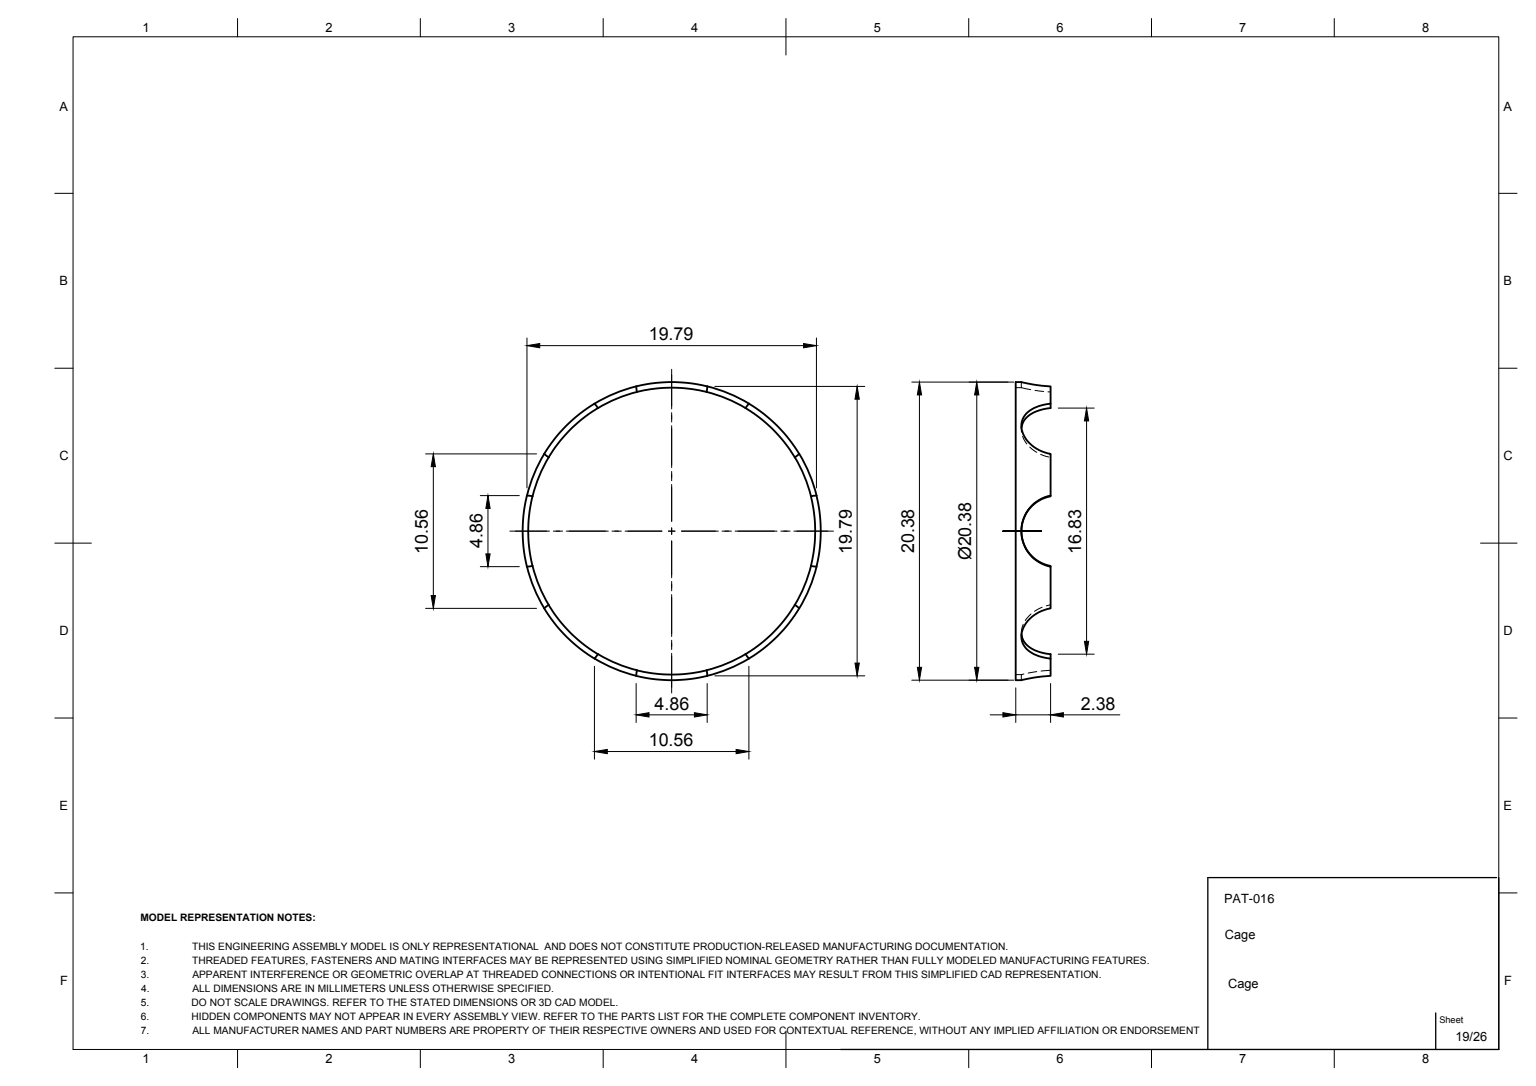
ISO-10303-21;
HEADER;
/* Generated by software containing ST-Developer
 * from STEP Tools, Inc. (www.steptools.com) 
 */

FILE_DESCRIPTION(
/* description */ ('Bracket-mounted idler roller'),
/* implementation_level */ '2;1');

FILE_NAME(
/* name */ 'Cage.step',
/* time_stamp */ '2026-10-28T03:26:42-07:00',
/* author */ (''),
/* organization */ (''),
/* preprocessor_version */ 'ST-DEVELOPER v20.2',
/* originating_system */ 'Autodesk Translation Framework v15.17.0.0',
/* authorisation */ '');

FILE_SCHEMA (('AUTOMOTIVE_DESIGN { 1 0 10303 214 3 1 1 }'));
ENDSEC;

DATA;
#10=MECHANICAL_DESIGN_GEOMETRIC_PRESENTATION_REPRESENTATION('',(#301),#6241);
#187=B_SPLINE_CURVE_WITH_KNOTS('',3,(#5456,#5457,#5458,#5459,#5460,#5461,
#5462,#5463,#5464,#5465,#5466,#5467,#5468,#5469,#5470,#5471,#5472,#5473,
#5474,#5475,#5476,#5477),.UNSPECIFIED.,.F.,.F.,(4,2,2,2,2,2,2,2,2,2,4),
(0.0473477652366656,0.126350602536658,0.189525903804987,0.252701205073317,
0.313298422430275,0.373895639787233,0.434492857144191,0.495090074501149,
0.558265375769478,0.621440677037807,0.7004435143378),.UNSPECIFIED.);
#188=B_SPLINE_CURVE_WITH_KNOTS('',3,(#5481,#5482,#5483,#5484,#5485,#5486,
#5487,#5488,#5489,#5490,#5491,#5492,#5493,#5494,#5495,#5496,#5497,#5498,
#5499,#5500,#5501,#5502),.UNSPECIFIED.,.F.,.F.,(4,2,2,2,2,2,2,2,2,2,4),
(0.0464897534940957,0.0852567806515119,0.170513561303024,0.246687263103517,
0.308657850341199,0.370628437578881,0.432599024816563,0.494569612054245,
0.570743313854739,0.656000094506251,0.694767121663666),.UNSPECIFIED.);
#189=B_SPLINE_CURVE_WITH_KNOTS('',3,(#5508,#5509,#5510,#5511,#5512,#5513,
#5514,#5515,#5516,#5517,#5518,#5519,#5520,#5521,#5522,#5523,#5524,#5525,
#5526,#5527,#5528,#5529),.UNSPECIFIED.,.F.,.F.,(4,2,2,2,2,2,2,2,2,2,4),
(0.0464897534940957,0.0852567806515118,0.170513561303024,0.246687263103517,
0.308657850341199,0.370628437578881,0.432599024816563,0.494569612054245,
0.570743313854738,0.65600009450625,0.694767121663666),.UNSPECIFIED.);
#190=B_SPLINE_CURVE_WITH_KNOTS('',3,(#5533,#5534,#5535,#5536,#5537,#5538,
#5539,#5540,#5541,#5542,#5543,#5544,#5545,#5546,#5547,#5548,#5549,#5550,
#5551,#5552,#5553,#5554),.UNSPECIFIED.,.F.,.F.,(4,2,2,2,2,2,2,2,2,2,4),
(0.0464897534940957,0.0852567806515119,0.170513561303024,0.246687263103517,
0.308657850341199,0.370628437578881,0.432599024816563,0.494569612054245,
0.570743313854739,0.656000094506251,0.694767121663666),.UNSPECIFIED.);
#191=B_SPLINE_CURVE_WITH_KNOTS('',3,(#5558,#5559,#5560,#5561,#5562,#5563,
#5564,#5565,#5566,#5567,#5568,#5569),.UNSPECIFIED.,.F.,.F.,(4,2,2,2,2,4),
(0.0464897534940957,0.0852567806515119,0.170513561303024,0.246687263103517,
0.308657850341199,0.370628437578881),.UNSPECIFIED.);
#192=B_SPLINE_CURVE_WITH_KNOTS('',3,(#5574,#5575,#5576,#5577,#5578,#5579,
#5580,#5581,#5582,#5583,#5584,#5585),.UNSPECIFIED.,.F.,.F.,(4,2,2,2,2,4),
(0.370628437578881,0.432599024816563,0.494569612054245,0.570743313854738,
0.65600009450625,0.694767121663666),.UNSPECIFIED.);
#193=B_SPLINE_CURVE_WITH_KNOTS('',3,(#5589,#5590,#5591,#5592,#5593,#5594,
#5595,#5596,#5597,#5598,#5599,#5600,#5601,#5602,#5603,#5604,#5605,#5606,
#5607,#5608,#5609,#5610),.UNSPECIFIED.,.F.,.F.,(4,2,2,2,2,2,2,2,2,2,4),
(0.0464897534940957,0.0852567806515121,0.170513561303024,0.246687263103518,
0.308657850341199,0.370628437578881,0.432599024816563,0.494569612054245,
0.570743313854738,0.65600009450625,0.694767121663666),.UNSPECIFIED.);
#194=B_SPLINE_CURVE_WITH_KNOTS('',3,(#5614,#5615,#5616,#5617,#5618,#5619,
#5620,#5621,#5622,#5623,#5624,#5625,#5626,#5627,#5628,#5629,#5630,#5631,
#5632,#5633,#5634,#5635),.UNSPECIFIED.,.F.,.F.,(4,2,2,2,2,2,2,2,2,2,4),
(0.0464897534940957,0.0852567806515119,0.170513561303024,0.246687263103517,
0.308657850341199,0.370628437578881,0.432599024816563,0.494569612054245,
0.570743313854738,0.65600009450625,0.694767121663667),.UNSPECIFIED.);
#195=B_SPLINE_CURVE_WITH_KNOTS('',3,(#5639,#5640,#5641,#5642,#5643,#5644,
#5645,#5646,#5647,#5648,#5649,#5650,#5651,#5652,#5653,#5654,#5655,#5656,
#5657,#5658,#5659,#5660),.UNSPECIFIED.,.F.,.F.,(4,2,2,2,2,2,2,2,2,2,4),
(0.0464897534940957,0.0852567806515119,0.170513561303024,0.246687263103517,
0.308657850341199,0.370628437578881,0.432599024816563,0.494569612054245,
0.570743313854738,0.65600009450625,0.694767121663666),.UNSPECIFIED.);
#196=B_SPLINE_CURVE_WITH_KNOTS('',3,(#5664,#5665,#5666,#5667,#5668,#5669,
#5670,#5671,#5672,#5673,#5674,#5675,#5676,#5677,#5678,#5679,#5680,#5681,
#5682,#5683,#5684,#5685),.UNSPECIFIED.,.F.,.F.,(4,2,2,2,2,2,2,2,2,2,4),
(0.0464897534940957,0.0852567806515119,0.170513561303024,0.246687263103517,
0.308657850341199,0.370628437578881,0.432599024816563,0.494569612054245,
0.570743313854739,0.656000094506251,0.694767121663667),.UNSPECIFIED.);
#197=B_SPLINE_CURVE_WITH_KNOTS('',3,(#5693,#5694,#5695,#5696,#5697,#5698,
#5699,#5700,#5701,#5702,#5703,#5704,#5705,#5706,#5707,#5708,#5709,#5710,
#5711,#5712,#5713,#5714),.UNSPECIFIED.,.F.,.F.,(4,2,2,2,2,2,2,2,2,2,4),
(0.0473477652366656,0.126350602536658,0.189525903804987,0.252701205073316,
0.313298422430274,0.373895639787232,0.434492857144191,0.495090074501149,
0.558265375769478,0.621440677037807,0.7004435143378),.UNSPECIFIED.);
#198=B_SPLINE_CURVE_WITH_KNOTS('',3,(#5722,#5723,#5724,#5725,#5726,#5727,
#5728,#5729,#5730,#5731,#5732,#5733,#5734,#5735,#5736,#5737,#5738,#5739,
#5740,#5741,#5742,#5743),.UNSPECIFIED.,.F.,.F.,(4,2,2,2,2,2,2,2,2,2,4),
(0.0473477652366656,0.126350602536658,0.189525903804987,0.252701205073317,
0.313298422430275,0.373895639787233,0.434492857144191,0.495090074501149,
0.558265375769478,0.621440677037807,0.7004435143378),.UNSPECIFIED.);
#199=B_SPLINE_CURVE_WITH_KNOTS('',3,(#5752,#5753,#5754,#5755,#5756,#5757,
#5758,#5759,#5760,#5761,#5762,#5763),.UNSPECIFIED.,.F.,.F.,(4,2,2,2,2,4),
(0.0473477652366656,0.126350602536658,0.189525903804987,0.252701205073316,
0.313298422430275,0.373895639787233),.UNSPECIFIED.);
#200=B_SPLINE_CURVE_WITH_KNOTS('',3,(#5765,#5766,#5767,#5768,#5769,#5770,
#5771,#5772,#5773,#5774,#5775,#5776),.UNSPECIFIED.,.F.,.F.,(4,2,2,2,2,4),
(0.373895639787233,0.434492857144191,0.495090074501149,0.558265375769478,
0.621440677037807,0.7004435143378),.UNSPECIFIED.);
#201=B_SPLINE_CURVE_WITH_KNOTS('',3,(#5783,#5784,#5785,#5786,#5787,#5788,
#5789,#5790,#5791,#5792,#5793,#5794,#5795,#5796,#5797,#5798,#5799,#5800,
#5801,#5802,#5803,#5804),.UNSPECIFIED.,.F.,.F.,(4,2,2,2,2,2,2,2,2,2,4),
(0.0473477652366656,0.126350602536658,0.189525903804987,0.252701205073316,
0.313298422430275,0.373895639787233,0.434492857144191,0.495090074501149,
0.558265375769478,0.621440677037807,0.7004435143378),.UNSPECIFIED.);
#202=B_SPLINE_CURVE_WITH_KNOTS('',3,(#5812,#5813,#5814,#5815,#5816,#5817,
#5818,#5819,#5820,#5821,#5822,#5823,#5824,#5825,#5826,#5827,#5828,#5829,
#5830,#5831,#5832,#5833),.UNSPECIFIED.,.F.,.F.,(4,2,2,2,2,2,2,2,2,2,4),
(0.0473477652366656,0.126350602536658,0.189525903804987,0.252701205073317,
0.313298422430275,0.373895639787233,0.434492857144191,0.495090074501149,
0.558265375769478,0.621440677037807,0.7004435143378),.UNSPECIFIED.);
#203=B_SPLINE_CURVE_WITH_KNOTS('',3,(#5841,#5842,#5843,#5844,#5845,#5846,
#5847,#5848,#5849,#5850,#5851,#5852,#5853,#5854,#5855,#5856,#5857,#5858,
#5859,#5860,#5861,#5862),.UNSPECIFIED.,.F.,.F.,(4,2,2,2,2,2,2,2,2,2,4),
(0.0473477652366656,0.126350602536658,0.189525903804987,0.252701205073316,
0.313298422430275,0.373895639787233,0.434492857144191,0.495090074501149,
0.558265375769478,0.621440677037807,0.7004435143378),.UNSPECIFIED.);
#204=B_SPLINE_CURVE_WITH_KNOTS('',3,(#5871,#5872,#5873,#5874,#5875,#5876,
#5877,#5878,#5879,#5880,#5881,#5882,#5883,#5884,#5885,#5886,#5887,#5888,
#5889,#5890,#5891,#5892),.UNSPECIFIED.,.F.,.F.,(4,2,2,2,2,2,2,2,2,2,4),
(0.0473477652366656,0.126350602536658,0.189525903804987,0.252701205073317,
0.313298422430275,0.373895639787233,0.434492857144191,0.495090074501149,
0.558265375769478,0.621440677037807,0.7004435143378),.UNSPECIFIED.);
#213=SPHERICAL_SURFACE('',#3665,0.247676);
#214=SPHERICAL_SURFACE('',#3681,0.247676);
#215=SPHERICAL_SURFACE('',#3686,0.247676);
#216=SPHERICAL_SURFACE('',#3691,0.247676);
#217=SPHERICAL_SURFACE('',#3696,0.247676);
#218=SPHERICAL_SURFACE('',#3701,0.247676);
#219=SPHERICAL_SURFACE('',#3706,0.247676);
#220=SPHERICAL_SURFACE('',#3714,0.247676);
#252=SHAPE_REPRESENTATION_RELATIONSHIP('SRR','None',#6357,#273);
#273=ADVANCED_BREP_SHAPE_REPRESENTATION('',(#329),#6233);
#301=STYLED_ITEM('',(#6538),#329);
#329=MANIFOLD_SOLID_BREP('Continuous crown cage',#3204);
#377=FACE_BOUND('',#881,.T.);
#482=PLANE('',#3678);
#483=PLANE('',#3683);
#484=PLANE('',#3688);
#485=PLANE('',#3693);
#486=PLANE('',#3698);
#487=PLANE('',#3703);
#488=PLANE('',#3712);
#489=PLANE('',#3716);
#490=PLANE('',#3717);
#631=FACE_OUTER_BOUND('',#863,.T.);
#632=FACE_OUTER_BOUND('',#864,.T.);
#633=FACE_OUTER_BOUND('',#865,.T.);
#634=FACE_OUTER_BOUND('',#866,.T.);
#635=FACE_OUTER_BOUND('',#867,.T.);
#636=FACE_OUTER_BOUND('',#868,.T.);
#637=FACE_OUTER_BOUND('',#869,.T.);
#638=FACE_OUTER_BOUND('',#870,.T.);
#639=FACE_OUTER_BOUND('',#871,.T.);
#640=FACE_OUTER_BOUND('',#872,.T.);
#641=FACE_OUTER_BOUND('',#873,.T.);
#642=FACE_OUTER_BOUND('',#874,.T.);
#643=FACE_OUTER_BOUND('',#875,.T.);
#644=FACE_OUTER_BOUND('',#876,.T.);
#645=FACE_OUTER_BOUND('',#877,.T.);
#646=FACE_OUTER_BOUND('',#878,.T.);
#647=FACE_OUTER_BOUND('',#879,.T.);
#648=FACE_OUTER_BOUND('',#880,.T.);
#649=FACE_OUTER_BOUND('',#882,.T.);
#863=EDGE_LOOP('',(#2600,#2601,#2602,#2603));
#864=EDGE_LOOP('',(#2604,#2605,#2606,#2607,#2608,#2609,#2610,#2611,#2612,
#2613,#2614,#2615,#2616,#2617,#2618,#2619,#2620,#2621,#2622,#2623));
#865=EDGE_LOOP('',(#2624,#2625,#2626,#2627));
#866=EDGE_LOOP('',(#2628,#2629,#2630,#2631));
#867=EDGE_LOOP('',(#2632,#2633,#2634,#2635));
#868=EDGE_LOOP('',(#2636,#2637,#2638,#2639));
#869=EDGE_LOOP('',(#2640,#2641,#2642,#2643));
#870=EDGE_LOOP('',(#2644,#2645,#2646,#2647,#2648,#2649));
#871=EDGE_LOOP('',(#2650,#2651,#2652,#2653));
#872=EDGE_LOOP('',(#2654,#2655,#2656,#2657));
#873=EDGE_LOOP('',(#2658,#2659,#2660,#2661));
#874=EDGE_LOOP('',(#2662,#2663,#2664,#2665));
#875=EDGE_LOOP('',(#2666,#2667,#2668,#2669));
#876=EDGE_LOOP('',(#2670,#2671,#2672,#2673));
#877=EDGE_LOOP('',(#2674,#2675,#2676,#2677,#2678,#2679,#2680,#2681,#2682,
#2683,#2684,#2685,#2686,#2687,#2688,#2689,#2690,#2691,#2692,#2693));
#878=EDGE_LOOP('',(#2694,#2695,#2696,#2697));
#879=EDGE_LOOP('',(#2698,#2699,#2700,#2701));
#880=EDGE_LOOP('',(#2702));
#881=EDGE_LOOP('',(#2703));
#882=EDGE_LOOP('',(#2704,#2705,#2706,#2707));
#1109=LINE('',#5571,#1291);
#1110=LINE('',#5867,#1292);
#1291=VECTOR('',#4470,1.019052);
#1292=VECTOR('',#4547,0.980948);
#1430=CIRCLE('',#3666,0.243053047864041);
#1431=CIRCLE('',#3667,0.243053047864041);
#1432=CIRCLE('',#3669,1.019052);
#1433=CIRCLE('',#3670,1.019052);
#1434=CIRCLE('',#3671,1.019052);
#1435=CIRCLE('',#3672,1.019052);
#1436=CIRCLE('',#3673,1.019052);
#1437=CIRCLE('',#3674,1.019052);
#1438=CIRCLE('',#3675,1.019052);
#1439=CIRCLE('',#3676,1.019052);
#1440=CIRCLE('',#3677,1.019052);
#1441=CIRCLE('',#3679,0.980948);
#1442=CIRCLE('',#3680,0.243053047864041);
#1443=CIRCLE('',#3682,0.243053047864041);
#1444=CIRCLE('',#3684,0.980948);
#1445=CIRCLE('',#3685,0.243053047864041);
#1446=CIRCLE('',#3687,0.243053047864041);
#1447=CIRCLE('',#3689,0.980948);
#1448=CIRCLE('',#3690,0.243053047864041);
#1449=CIRCLE('',#3692,0.243053047864041);
#1450=CIRCLE('',#3694,0.980948);
#1451=CIRCLE('',#3695,0.243053047864041);
#1452=CIRCLE('',#3697,0.243053047864041);
#1453=CIRCLE('',#3699,0.980948);
#1454=CIRCLE('',#3700,0.243053047864041);
#1455=CIRCLE('',#3702,0.243053047864041);
#1456=CIRCLE('',#3704,0.980948);
#1457=CIRCLE('',#3705,0.243053047864041);
#1458=CIRCLE('',#3707,0.243053047864041);
#1459=CIRCLE('',#3709,0.980948);
#1460=CIRCLE('',#3710,0.980948);
#1461=CIRCLE('',#3711,0.980948);
#1462=CIRCLE('',#3713,0.243053047864041);
#1463=CIRCLE('',#3715,0.243053047864041);
#1677=VERTEX_POINT('',#5454);
#1678=VERTEX_POINT('',#5455);
#1679=VERTEX_POINT('',#5478);
#1680=VERTEX_POINT('',#5480);
#1681=VERTEX_POINT('',#5505);
#1682=VERTEX_POINT('',#5507);
#1683=VERTEX_POINT('',#5530);
#1684=VERTEX_POINT('',#5532);
#1685=VERTEX_POINT('',#5555);
#1686=VERTEX_POINT('',#5557);
#1687=VERTEX_POINT('',#5570);
#1688=VERTEX_POINT('',#5573);
#1689=VERTEX_POINT('',#5586);
#1690=VERTEX_POINT('',#5588);
#1691=VERTEX_POINT('',#5611);
#1692=VERTEX_POINT('',#5613);
#1693=VERTEX_POINT('',#5636);
#1694=VERTEX_POINT('',#5638);
#1695=VERTEX_POINT('',#5661);
#1696=VERTEX_POINT('',#5663);
#1697=VERTEX_POINT('',#5688);
#1698=VERTEX_POINT('',#5692);
#1699=VERTEX_POINT('',#5717);
#1700=VERTEX_POINT('',#5721);
#1701=VERTEX_POINT('',#5746);
#1702=VERTEX_POINT('',#5750);
#1703=VERTEX_POINT('',#5751);
#1704=VERTEX_POINT('',#5778);
#1705=VERTEX_POINT('',#5782);
#1706=VERTEX_POINT('',#5807);
#1707=VERTEX_POINT('',#5811);
#1708=VERTEX_POINT('',#5836);
#1709=VERTEX_POINT('',#5840);
#1710=VERTEX_POINT('',#5865);
#1711=VERTEX_POINT('',#5868);
#1712=VERTEX_POINT('',#5870);
#2002=EDGE_CURVE('',#1677,#1678,#187,.T.);
#2003=EDGE_CURVE('',#1679,#1677,#1430,.T.);
#2004=EDGE_CURVE('',#1680,#1679,#188,.T.);
#2005=EDGE_CURVE('',#1678,#1680,#1431,.T.);
#2006=EDGE_CURVE('',#1681,#1679,#1432,.T.);
#2007=EDGE_CURVE('',#1681,#1682,#189,.T.);
#2008=EDGE_CURVE('',#1683,#1682,#1433,.T.);
#2009=EDGE_CURVE('',#1683,#1684,#190,.T.);
#2010=EDGE_CURVE('',#1685,#1684,#1434,.T.);
#2011=EDGE_CURVE('',#1685,#1686,#191,.T.);
#2012=EDGE_CURVE('',#1686,#1687,#1109,.T.);
#2013=EDGE_CURVE('',#1687,#1687,#1435,.T.);
#2014=EDGE_CURVE('',#1686,#1688,#192,.T.);
#2015=EDGE_CURVE('',#1689,#1688,#1436,.T.);
#2016=EDGE_CURVE('',#1689,#1690,#193,.T.);
#2017=EDGE_CURVE('',#1691,#1690,#1437,.T.);
#2018=EDGE_CURVE('',#1691,#1692,#194,.T.);
#2019=EDGE_CURVE('',#1693,#1692,#1438,.T.);
#2020=EDGE_CURVE('',#1693,#1694,#195,.T.);
#2021=EDGE_CURVE('',#1695,#1694,#1439,.T.);
#2022=EDGE_CURVE('',#1695,#1696,#196,.T.);
#2023=EDGE_CURVE('',#1680,#1696,#1440,.T.);
#2024=EDGE_CURVE('',#1677,#1697,#1441,.T.);
#2025=EDGE_CURVE('',#1697,#1681,#1442,.T.);
#2026=EDGE_CURVE('',#1698,#1697,#197,.T.);
#2027=EDGE_CURVE('',#1682,#1698,#1443,.T.);
#2028=EDGE_CURVE('',#1698,#1699,#1444,.T.);
#2029=EDGE_CURVE('',#1699,#1683,#1445,.T.);
#2030=EDGE_CURVE('',#1700,#1699,#198,.T.);
#2031=EDGE_CURVE('',#1684,#1700,#1446,.T.);
#2032=EDGE_CURVE('',#1700,#1701,#1447,.T.);
#2033=EDGE_CURVE('',#1701,#1685,#1448,.T.);
#2034=EDGE_CURVE('',#1702,#1703,#199,.T.);
#2035=EDGE_CURVE('',#1688,#1702,#1449,.T.);
#2036=EDGE_CURVE('',#1703,#1701,#200,.T.);
#2037=EDGE_CURVE('',#1702,#1704,#1450,.T.);
#2038=EDGE_CURVE('',#1704,#1689,#1451,.T.);
#2039=EDGE_CURVE('',#1705,#1704,#201,.T.);
#2040=EDGE_CURVE('',#1690,#1705,#1452,.T.);
#2041=EDGE_CURVE('',#1705,#1706,#1453,.T.);
#2042=EDGE_CURVE('',#1706,#1691,#1454,.T.);
#2043=EDGE_CURVE('',#1707,#1706,#202,.T.);
#2044=EDGE_CURVE('',#1692,#1707,#1455,.T.);
#2045=EDGE_CURVE('',#1707,#1708,#1456,.T.);
#2046=EDGE_CURVE('',#1708,#1693,#1457,.T.);
#2047=EDGE_CURVE('',#1709,#1708,#203,.T.);
#2048=EDGE_CURVE('',#1694,#1709,#1458,.T.);
#2049=EDGE_CURVE('',#1710,#1710,#1459,.T.);
#2050=EDGE_CURVE('',#1710,#1703,#1110,.T.);
#2051=EDGE_CURVE('',#1711,#1678,#1460,.T.);
#2052=EDGE_CURVE('',#1711,#1712,#204,.T.);
#2053=EDGE_CURVE('',#1709,#1712,#1461,.T.);
#2054=EDGE_CURVE('',#1696,#1711,#1462,.T.);
#2055=EDGE_CURVE('',#1712,#1695,#1463,.T.);
#2600=ORIENTED_EDGE('',*,*,#2002,.F.);
#2601=ORIENTED_EDGE('',*,*,#2003,.F.);
#2602=ORIENTED_EDGE('',*,*,#2004,.F.);
#2603=ORIENTED_EDGE('',*,*,#2005,.F.);
#2604=ORIENTED_EDGE('',*,*,#2004,.T.);
#2605=ORIENTED_EDGE('',*,*,#2006,.F.);
#2606=ORIENTED_EDGE('',*,*,#2007,.T.);
#2607=ORIENTED_EDGE('',*,*,#2008,.F.);
#2608=ORIENTED_EDGE('',*,*,#2009,.T.);
#2609=ORIENTED_EDGE('',*,*,#2010,.F.);
#2610=ORIENTED_EDGE('',*,*,#2011,.T.);
#2611=ORIENTED_EDGE('',*,*,#2012,.T.);
#2612=ORIENTED_EDGE('',*,*,#2013,.F.);
#2613=ORIENTED_EDGE('',*,*,#2012,.F.);
#2614=ORIENTED_EDGE('',*,*,#2014,.T.);
#2615=ORIENTED_EDGE('',*,*,#2015,.F.);
#2616=ORIENTED_EDGE('',*,*,#2016,.T.);
#2617=ORIENTED_EDGE('',*,*,#2017,.F.);
#2618=ORIENTED_EDGE('',*,*,#2018,.T.);
#2619=ORIENTED_EDGE('',*,*,#2019,.F.);
#2620=ORIENTED_EDGE('',*,*,#2020,.T.);
#2621=ORIENTED_EDGE('',*,*,#2021,.F.);
#2622=ORIENTED_EDGE('',*,*,#2022,.T.);
#2623=ORIENTED_EDGE('',*,*,#2023,.F.);
#2624=ORIENTED_EDGE('',*,*,#2003,.T.);
#2625=ORIENTED_EDGE('',*,*,#2024,.T.);
#2626=ORIENTED_EDGE('',*,*,#2025,.T.);
#2627=ORIENTED_EDGE('',*,*,#2006,.T.);
#2628=ORIENTED_EDGE('',*,*,#2026,.F.);
#2629=ORIENTED_EDGE('',*,*,#2027,.F.);
#2630=ORIENTED_EDGE('',*,*,#2007,.F.);
#2631=ORIENTED_EDGE('',*,*,#2025,.F.);
#2632=ORIENTED_EDGE('',*,*,#2027,.T.);
#2633=ORIENTED_EDGE('',*,*,#2028,.T.);
#2634=ORIENTED_EDGE('',*,*,#2029,.T.);
#2635=ORIENTED_EDGE('',*,*,#2008,.T.);
#2636=ORIENTED_EDGE('',*,*,#2030,.F.);
#2637=ORIENTED_EDGE('',*,*,#2031,.F.);
#2638=ORIENTED_EDGE('',*,*,#2009,.F.);
#2639=ORIENTED_EDGE('',*,*,#2029,.F.);
#2640=ORIENTED_EDGE('',*,*,#2031,.T.);
#2641=ORIENTED_EDGE('',*,*,#2032,.T.);
#2642=ORIENTED_EDGE('',*,*,#2033,.T.);
#2643=ORIENTED_EDGE('',*,*,#2010,.T.);
#2644=ORIENTED_EDGE('',*,*,#2034,.F.);
#2645=ORIENTED_EDGE('',*,*,#2035,.F.);
#2646=ORIENTED_EDGE('',*,*,#2014,.F.);
#2647=ORIENTED_EDGE('',*,*,#2011,.F.);
#2648=ORIENTED_EDGE('',*,*,#2033,.F.);
#2649=ORIENTED_EDGE('',*,*,#2036,.F.);
#2650=ORIENTED_EDGE('',*,*,#2035,.T.);
#2651=ORIENTED_EDGE('',*,*,#2037,.T.);
#2652=ORIENTED_EDGE('',*,*,#2038,.T.);
#2653=ORIENTED_EDGE('',*,*,#2015,.T.);
#2654=ORIENTED_EDGE('',*,*,#2039,.F.);
#2655=ORIENTED_EDGE('',*,*,#2040,.F.);
#2656=ORIENTED_EDGE('',*,*,#2016,.F.);
#2657=ORIENTED_EDGE('',*,*,#2038,.F.);
#2658=ORIENTED_EDGE('',*,*,#2040,.T.);
#2659=ORIENTED_EDGE('',*,*,#2041,.T.);
#2660=ORIENTED_EDGE('',*,*,#2042,.T.);
#2661=ORIENTED_EDGE('',*,*,#2017,.T.);
#2662=ORIENTED_EDGE('',*,*,#2043,.F.);
#2663=ORIENTED_EDGE('',*,*,#2044,.F.);
#2664=ORIENTED_EDGE('',*,*,#2018,.F.);
#2665=ORIENTED_EDGE('',*,*,#2042,.F.);
#2666=ORIENTED_EDGE('',*,*,#2044,.T.);
#2667=ORIENTED_EDGE('',*,*,#2045,.T.);
#2668=ORIENTED_EDGE('',*,*,#2046,.T.);
#2669=ORIENTED_EDGE('',*,*,#2019,.T.);
#2670=ORIENTED_EDGE('',*,*,#2020,.F.);
#2671=ORIENTED_EDGE('',*,*,#2046,.F.);
#2672=ORIENTED_EDGE('',*,*,#2047,.F.);
#2673=ORIENTED_EDGE('',*,*,#2048,.F.);
#2674=ORIENTED_EDGE('',*,*,#2049,.F.);
#2675=ORIENTED_EDGE('',*,*,#2050,.T.);
#2676=ORIENTED_EDGE('',*,*,#2036,.T.);
#2677=ORIENTED_EDGE('',*,*,#2032,.F.);
#2678=ORIENTED_EDGE('',*,*,#2030,.T.);
#2679=ORIENTED_EDGE('',*,*,#2028,.F.);
#2680=ORIENTED_EDGE('',*,*,#2026,.T.);
#2681=ORIENTED_EDGE('',*,*,#2024,.F.);
#2682=ORIENTED_EDGE('',*,*,#2002,.T.);
#2683=ORIENTED_EDGE('',*,*,#2051,.F.);
#2684=ORIENTED_EDGE('',*,*,#2052,.T.);
#2685=ORIENTED_EDGE('',*,*,#2053,.F.);
#2686=ORIENTED_EDGE('',*,*,#2047,.T.);
#2687=ORIENTED_EDGE('',*,*,#2045,.F.);
#2688=ORIENTED_EDGE('',*,*,#2043,.T.);
#2689=ORIENTED_EDGE('',*,*,#2041,.F.);
#2690=ORIENTED_EDGE('',*,*,#2039,.T.);
#2691=ORIENTED_EDGE('',*,*,#2037,.F.);
#2692=ORIENTED_EDGE('',*,*,#2034,.T.);
#2693=ORIENTED_EDGE('',*,*,#2050,.F.);
#2694=ORIENTED_EDGE('',*,*,#2005,.T.);
#2695=ORIENTED_EDGE('',*,*,#2023,.T.);
#2696=ORIENTED_EDGE('',*,*,#2054,.T.);
#2697=ORIENTED_EDGE('',*,*,#2051,.T.);
#2698=ORIENTED_EDGE('',*,*,#2022,.F.);
#2699=ORIENTED_EDGE('',*,*,#2055,.F.);
#2700=ORIENTED_EDGE('',*,*,#2052,.F.);
#2701=ORIENTED_EDGE('',*,*,#2054,.F.);
#2702=ORIENTED_EDGE('',*,*,#2013,.T.);
#2703=ORIENTED_EDGE('',*,*,#2049,.T.);
#2704=ORIENTED_EDGE('',*,*,#2048,.T.);
#2705=ORIENTED_EDGE('',*,*,#2053,.T.);
#2706=ORIENTED_EDGE('',*,*,#2055,.T.);
#2707=ORIENTED_EDGE('',*,*,#2021,.T.);
#2961=CYLINDRICAL_SURFACE('',#3668,1.019052);
#2962=CYLINDRICAL_SURFACE('',#3708,0.980948);
#3106=ADVANCED_FACE('',(#631),#213,.F.);
#3107=ADVANCED_FACE('',(#632),#2961,.T.);
#3108=ADVANCED_FACE('',(#633),#482,.T.);
#3109=ADVANCED_FACE('',(#634),#214,.F.);
#3110=ADVANCED_FACE('',(#635),#483,.T.);
#3111=ADVANCED_FACE('',(#636),#215,.F.);
#3112=ADVANCED_FACE('',(#637),#484,.T.);
#3113=ADVANCED_FACE('',(#638),#216,.F.);
#3114=ADVANCED_FACE('',(#639),#485,.T.);
#3115=ADVANCED_FACE('',(#640),#217,.F.);
#3116=ADVANCED_FACE('',(#641),#486,.T.);
#3117=ADVANCED_FACE('',(#642),#218,.F.);
#3118=ADVANCED_FACE('',(#643),#487,.T.);
#3119=ADVANCED_FACE('',(#644),#219,.F.);
#3120=ADVANCED_FACE('',(#645),#2962,.F.);
#3121=ADVANCED_FACE('',(#646),#488,.T.);
#3122=ADVANCED_FACE('',(#647),#220,.F.);
#3123=ADVANCED_FACE('',(#648,#377),#489,.T.);
#3124=ADVANCED_FACE('',(#649),#490,.T.);
#3204=CLOSED_SHELL('',(#3106,#3107,#3108,#3109,#3110,#3111,#3112,#3113,
#3114,#3115,#3116,#3117,#3118,#3119,#3120,#3121,#3122,#3123,#3124));
#3664=AXIS2_PLACEMENT_3D('',#5452,#4454,#4455);
#3665=AXIS2_PLACEMENT_3D('',#5453,#4456,#4457);
#3666=AXIS2_PLACEMENT_3D('',#5479,#4458,#4459);
#3667=AXIS2_PLACEMENT_3D('',#5503,#4460,#4461);
#3668=AXIS2_PLACEMENT_3D('',#5504,#4462,#4463);
#3669=AXIS2_PLACEMENT_3D('',#5506,#4464,#4465);
#3670=AXIS2_PLACEMENT_3D('',#5531,#4466,#4467);
#3671=AXIS2_PLACEMENT_3D('',#5556,#4468,#4469);
#3672=AXIS2_PLACEMENT_3D('',#5572,#4471,#4472);
#3673=AXIS2_PLACEMENT_3D('',#5587,#4473,#4474);
#3674=AXIS2_PLACEMENT_3D('',#5612,#4475,#4476);
#3675=AXIS2_PLACEMENT_3D('',#5637,#4477,#4478);
#3676=AXIS2_PLACEMENT_3D('',#5662,#4479,#4480);
#3677=AXIS2_PLACEMENT_3D('',#5686,#4481,#4482);
#3678=AXIS2_PLACEMENT_3D('',#5687,#4483,#4484);
#3679=AXIS2_PLACEMENT_3D('',#5689,#4485,#4486);
#3680=AXIS2_PLACEMENT_3D('',#5690,#4487,#4488);
#3681=AXIS2_PLACEMENT_3D('',#5691,#4489,#4490);
#3682=AXIS2_PLACEMENT_3D('',#5715,#4491,#4492);
#3683=AXIS2_PLACEMENT_3D('',#5716,#4493,#4494);
#3684=AXIS2_PLACEMENT_3D('',#5718,#4495,#4496);
#3685=AXIS2_PLACEMENT_3D('',#5719,#4497,#4498);
#3686=AXIS2_PLACEMENT_3D('',#5720,#4499,#4500);
#3687=AXIS2_PLACEMENT_3D('',#5744,#4501,#4502);
#3688=AXIS2_PLACEMENT_3D('',#5745,#4503,#4504);
#3689=AXIS2_PLACEMENT_3D('',#5747,#4505,#4506);
#3690=AXIS2_PLACEMENT_3D('',#5748,#4507,#4508);
#3691=AXIS2_PLACEMENT_3D('',#5749,#4509,#4510);
#3692=AXIS2_PLACEMENT_3D('',#5764,#4511,#4512);
#3693=AXIS2_PLACEMENT_3D('',#5777,#4513,#4514);
#3694=AXIS2_PLACEMENT_3D('',#5779,#4515,#4516);
#3695=AXIS2_PLACEMENT_3D('',#5780,#4517,#4518);
#3696=AXIS2_PLACEMENT_3D('',#5781,#4519,#4520);
#3697=AXIS2_PLACEMENT_3D('',#5805,#4521,#4522);
#3698=AXIS2_PLACEMENT_3D('',#5806,#4523,#4524);
#3699=AXIS2_PLACEMENT_3D('',#5808,#4525,#4526);
#3700=AXIS2_PLACEMENT_3D('',#5809,#4527,#4528);
#3701=AXIS2_PLACEMENT_3D('',#5810,#4529,#4530);
#3702=AXIS2_PLACEMENT_3D('',#5834,#4531,#4532);
#3703=AXIS2_PLACEMENT_3D('',#5835,#4533,#4534);
#3704=AXIS2_PLACEMENT_3D('',#5837,#4535,#4536);
#3705=AXIS2_PLACEMENT_3D('',#5838,#4537,#4538);
#3706=AXIS2_PLACEMENT_3D('',#5839,#4539,#4540);
#3707=AXIS2_PLACEMENT_3D('',#5863,#4541,#4542);
#3708=AXIS2_PLACEMENT_3D('',#5864,#4543,#4544);
#3709=AXIS2_PLACEMENT_3D('',#5866,#4545,#4546);
#3710=AXIS2_PLACEMENT_3D('',#5869,#4548,#4549);
#3711=AXIS2_PLACEMENT_3D('',#5893,#4550,#4551);
#3712=AXIS2_PLACEMENT_3D('',#5894,#4552,#4553);
#3713=AXIS2_PLACEMENT_3D('',#5895,#4554,#4555);
#3714=AXIS2_PLACEMENT_3D('',#5896,#4556,#4557);
#3715=AXIS2_PLACEMENT_3D('',#5897,#4558,#4559);
#3716=AXIS2_PLACEMENT_3D('',#5898,#4560,#4561);
#3717=AXIS2_PLACEMENT_3D('',#5899,#4562,#4563);
#4454=DIRECTION('axis',(0.,0.,1.));
#4455=DIRECTION('refdir',(1.,0.,0.));
#4456=DIRECTION('center_axis',(0.,0.,1.));
#4457=DIRECTION('ref_axis',(1.,0.,0.));
#4458=DIRECTION('center_axis',(0.,-1.,0.));
#4459=DIRECTION('ref_axis',(0.,0.,-1.));
#4460=DIRECTION('center_axis',(0.,-1.,0.));
#4461=DIRECTION('ref_axis',(0.,0.,-1.));
#4462=DIRECTION('center_axis',(0.,1.,0.));
#4463=DIRECTION('ref_axis',(1.,0.,0.));
#4464=DIRECTION('center_axis',(0.,1.,0.));
#4465=DIRECTION('ref_axis',(1.,0.,0.));
#4466=DIRECTION('center_axis',(0.,1.,0.));
#4467=DIRECTION('ref_axis',(1.,0.,0.));
#4468=DIRECTION('center_axis',(0.,1.,0.));
#4469=DIRECTION('ref_axis',(1.,0.,0.));
#4470=DIRECTION('',(0.,-1.,0.));
#4471=DIRECTION('center_axis',(0.,-1.,0.));
#4472=DIRECTION('ref_axis',(1.,0.,0.));
#4473=DIRECTION('center_axis',(0.,1.,0.));
#4474=DIRECTION('ref_axis',(1.,0.,0.));
#4475=DIRECTION('center_axis',(0.,1.,0.));
#4476=DIRECTION('ref_axis',(1.,0.,0.));
#4477=DIRECTION('center_axis',(0.,1.,0.));
#4478=DIRECTION('ref_axis',(1.,0.,0.));
#4479=DIRECTION('center_axis',(0.,1.,0.));
#4480=DIRECTION('ref_axis',(1.,0.,0.));
#4481=DIRECTION('center_axis',(0.,1.,0.));
#4482=DIRECTION('ref_axis',(1.,0.,0.));
#4483=DIRECTION('center_axis',(0.,1.,0.));
#4484=DIRECTION('ref_axis',(1.,0.,0.));
#4485=DIRECTION('center_axis',(0.,-1.,0.));
#4486=DIRECTION('ref_axis',(1.,0.,0.));
#4487=DIRECTION('center_axis',(0.,-1.,0.));
#4488=DIRECTION('ref_axis',(0.,0.,-1.));
#4489=DIRECTION('center_axis',(6.12323399573677E-17,0.,1.));
#4490=DIRECTION('ref_axis',(1.,0.,0.));
#4491=DIRECTION('center_axis',(0.,-1.,0.));
#4492=DIRECTION('ref_axis',(0.,0.,-1.));
#4493=DIRECTION('center_axis',(0.,1.,0.));
#4494=DIRECTION('ref_axis',(1.,0.,0.));
#4495=DIRECTION('center_axis',(0.,-1.,0.));
#4496=DIRECTION('ref_axis',(1.,0.,0.));
#4497=DIRECTION('center_axis',(0.,-1.,0.));
#4498=DIRECTION('ref_axis',(0.,0.,-1.));
#4499=DIRECTION('center_axis',(0.,0.,1.));
#4500=DIRECTION('ref_axis',(1.,0.,0.));
#4501=DIRECTION('center_axis',(0.,-1.,0.));
#4502=DIRECTION('ref_axis',(0.,0.,-1.));
#4503=DIRECTION('center_axis',(0.,1.,0.));
#4504=DIRECTION('ref_axis',(1.,0.,0.));
#4505=DIRECTION('center_axis',(0.,-1.,0.));
#4506=DIRECTION('ref_axis',(1.,0.,0.));
#4507=DIRECTION('center_axis',(0.,-1.,0.));
#4508=DIRECTION('ref_axis',(0.,0.,-1.));
#4509=DIRECTION('center_axis',(0.,0.,1.));
#4510=DIRECTION('ref_axis',(1.,0.,0.));
#4511=DIRECTION('center_axis',(0.,-1.,0.));
#4512=DIRECTION('ref_axis',(0.,0.,-1.));
#4513=DIRECTION('center_axis',(0.,1.,0.));
#4514=DIRECTION('ref_axis',(1.,0.,0.));
#4515=DIRECTION('center_axis',(0.,-1.,0.));
#4516=DIRECTION('ref_axis',(1.,0.,0.));
#4517=DIRECTION('center_axis',(0.,-1.,0.));
#4518=DIRECTION('ref_axis',(0.,0.,-1.));
#4519=DIRECTION('center_axis',(0.,0.,1.));
#4520=DIRECTION('ref_axis',(1.,0.,0.));
#4521=DIRECTION('center_axis',(0.,-1.,0.));
#4522=DIRECTION('ref_axis',(0.,0.,-1.));
#4523=DIRECTION('center_axis',(0.,1.,0.));
#4524=DIRECTION('ref_axis',(1.,0.,0.));
#4525=DIRECTION('center_axis',(0.,-1.,0.));
#4526=DIRECTION('ref_axis',(1.,0.,0.));
#4527=DIRECTION('center_axis',(0.,-1.,0.));
#4528=DIRECTION('ref_axis',(0.,0.,-1.));
#4529=DIRECTION('center_axis',(6.12323399573676E-17,0.,1.));
#4530=DIRECTION('ref_axis',(1.,0.,0.));
#4531=DIRECTION('center_axis',(0.,-1.,0.));
#4532=DIRECTION('ref_axis',(0.,0.,-1.));
#4533=DIRECTION('center_axis',(0.,1.,0.));
#4534=DIRECTION('ref_axis',(1.,0.,0.));
#4535=DIRECTION('center_axis',(0.,-1.,0.));
#4536=DIRECTION('ref_axis',(1.,0.,0.));
#4537=DIRECTION('center_axis',(0.,-1.,0.));
#4538=DIRECTION('ref_axis',(0.,0.,-1.));
#4539=DIRECTION('center_axis',(0.,0.,1.));
#4540=DIRECTION('ref_axis',(1.,0.,0.));
#4541=DIRECTION('center_axis',(0.,-1.,0.));
#4542=DIRECTION('ref_axis',(0.,0.,-1.));
#4543=DIRECTION('center_axis',(0.,1.,0.));
#4544=DIRECTION('ref_axis',(1.,0.,0.));
#4545=DIRECTION('center_axis',(0.,1.,0.));
#4546=DIRECTION('ref_axis',(1.,0.,0.));
#4547=DIRECTION('',(0.,1.,0.));
#4548=DIRECTION('center_axis',(0.,-1.,0.));
#4549=DIRECTION('ref_axis',(1.,0.,0.));
#4550=DIRECTION('center_axis',(0.,-1.,0.));
#4551=DIRECTION('ref_axis',(1.,0.,0.));
#4552=DIRECTION('center_axis',(0.,1.,0.));
#4553=DIRECTION('ref_axis',(1.,0.,0.));
#4554=DIRECTION('center_axis',(0.,-1.,0.));
#4555=DIRECTION('ref_axis',(0.,0.,-1.));
#4556=DIRECTION('center_axis',(0.,0.,1.));
#4557=DIRECTION('ref_axis',(1.,0.,0.));
#4558=DIRECTION('center_axis',(0.,-1.,0.));
#4559=DIRECTION('ref_axis',(0.,0.,-1.));
#4560=DIRECTION('center_axis',(0.,-1.,0.));
#4561=DIRECTION('ref_axis',(-1.,0.,0.));
#4562=DIRECTION('center_axis',(0.,1.,0.));
#4563=DIRECTION('ref_axis',(1.,0.,0.));
#5452=CARTESIAN_POINT('',(0.,0.,0.));
#5453=CARTESIAN_POINT('Origin',(0.707106781186547,0.,0.707106781186548));
#5454=CARTESIAN_POINT('',(0.504455939115715,-0.04763,0.841298510752802));
#5455=CARTESIAN_POINT('',(0.841298510752802,-0.04763,0.504455939115715));
#5456=CARTESIAN_POINT('Ctrl Pts',(0.504455939115715,-0.04763,0.841298510752802));
#5457=CARTESIAN_POINT('Ctrl Pts',(0.508899795931835,-0.0740444353928835,
0.838633903678357));
#5458=CARTESIAN_POINT('Ctrl Pts',(0.517157748491652,-0.0999305678883309,
0.833661031856294));
#5459=CARTESIAN_POINT('Ctrl Pts',(0.537715343527944,-0.142345102874864,
0.820511285096538));
#5460=CARTESIAN_POINT('Ctrl Pts',(0.548874290046456,-0.159766064500479,
0.813159949759));
#5461=CARTESIAN_POINT('Ctrl Pts',(0.573915184558107,-0.190326085855194,
0.795684265985089));
#5462=CARTESIAN_POINT('Ctrl Pts',(0.587792702767295,-0.203463743702801,
0.78555112003688));
#5463=CARTESIAN_POINT('Ctrl Pts',(0.615966552324775,-0.224161999508995,
0.763642258217233));
#5464=CARTESIAN_POINT('Ctrl Pts',(0.631684198665438,-0.232861760990032,
0.750785745543687));
#5465=CARTESIAN_POINT('Ctrl Pts',(0.663382628119203,-0.244251601209411,
0.722929908501543));
#5466=CARTESIAN_POINT('Ctrl Pts',(0.679352081686668,-0.246942143572133,
0.707917883896095));
#5467=CARTESIAN_POINT('Ctrl Pts',(0.707917883896095,-0.246942143572133,
0.679352081686668));
#5468=CARTESIAN_POINT('Ctrl Pts',(0.722929908501543,-0.244251601209411,
0.663382628119203));
#5469=CARTESIAN_POINT('Ctrl Pts',(0.750785745543687,-0.232861760990032,
0.631684198665439));
#5470=CARTESIAN_POINT('Ctrl Pts',(0.763642258217232,-0.224161999508995,
0.615966552324775));
#5471=CARTESIAN_POINT('Ctrl Pts',(0.78555112003688,-0.203463743702801,0.587792702767295));
#5472=CARTESIAN_POINT('Ctrl Pts',(0.795684265985088,-0.190326085855194,
0.573915184558108));
#5473=CARTESIAN_POINT('Ctrl Pts',(0.813159949759,-0.15976606450048,0.548874290046456));
#5474=CARTESIAN_POINT('Ctrl Pts',(0.820511285096538,-0.142345102874864,
0.537715343527944));
#5475=CARTESIAN_POINT('Ctrl Pts',(0.833661031856294,-0.099930567888331,
0.517157748491653));
#5476=CARTESIAN_POINT('Ctrl Pts',(0.838633903678357,-0.0740444353928835,
0.508899795931835));
#5477=CARTESIAN_POINT('Ctrl Pts',(0.841298510752801,-0.0476299999999999,
0.504455939115715));
#5478=CARTESIAN_POINT('',(0.528110872004958,-0.04763,0.871530771444223));
#5479=CARTESIAN_POINT('Origin',(0.707106781186547,-0.04763,0.707106781186548));
#5480=CARTESIAN_POINT('',(0.871530771444223,-0.04763,0.528110872004959));
#5481=CARTESIAN_POINT('Ctrl Pts',(0.871530771444223,-0.0476300000000001,
0.528110872004958));
#5482=CARTESIAN_POINT('Ctrl Pts',(0.87014664509073,-0.0609922781173483,
0.530395067942936));
#5483=CARTESIAN_POINT('Ctrl Pts',(0.868149331745851,-0.0742967091364493,
0.533674141594226));
#5484=CARTESIAN_POINT('Ctrl Pts',(0.85981294420286,-0.115492077056649,0.54708917182331));
#5485=CARTESIAN_POINT('Ctrl Pts',(0.850993704737257,-0.141695629206859,
0.560922177770136));
#5486=CARTESIAN_POINT('Ctrl Pts',(0.830754510485543,-0.181890537957859,
0.590422647829571));
#5487=CARTESIAN_POINT('Ctrl Pts',(0.816896541396381,-0.201072148666545,
0.609616703125488));
#5488=CARTESIAN_POINT('Ctrl Pts',(0.792310597819928,-0.223955109275652,
0.641117951819998));
#5489=CARTESIAN_POINT('Ctrl Pts',(0.779109323683612,-0.232742381310829,
0.657208095763053));
#5490=CARTESIAN_POINT('Ctrl Pts',(0.750552691816206,-0.244234834628584,
0.68964083160521));
#5491=CARTESIAN_POINT('Ctrl Pts',(0.735185187071673,-0.246942143572133,
0.705971972091755));
#5492=CARTESIAN_POINT('Ctrl Pts',(0.705971972091754,-0.246942143572133,
0.735185187071673));
#5493=CARTESIAN_POINT('Ctrl Pts',(0.689640831605209,-0.244234834628584,
0.750552691816206));
#5494=CARTESIAN_POINT('Ctrl Pts',(0.657208095763052,-0.232742381310829,
0.779109323683612));
#5495=CARTESIAN_POINT('Ctrl Pts',(0.641117951819998,-0.223955109275652,
0.792310597819928));
#5496=CARTESIAN_POINT('Ctrl Pts',(0.609616703125487,-0.201072148666545,
0.816896541396382));
#5497=CARTESIAN_POINT('Ctrl Pts',(0.590422647829571,-0.181890537957858,
0.830754510485544));
#5498=CARTESIAN_POINT('Ctrl Pts',(0.560922177770135,-0.141695629206858,
0.850993704737257));
#5499=CARTESIAN_POINT('Ctrl Pts',(0.547089171823309,-0.115492077056649,
0.859812944202861));
#5500=CARTESIAN_POINT('Ctrl Pts',(0.533674141594226,-0.0742967091364491,
0.868149331745852));
#5501=CARTESIAN_POINT('Ctrl Pts',(0.530395067942936,-0.0609922781173483,
0.870146645090731));
#5502=CARTESIAN_POINT('Ctrl Pts',(0.528110872004958,-0.0476300000000001,
0.871530771444223));
#5503=CARTESIAN_POINT('Origin',(0.707106781186547,-0.04763,0.707106781186548));
#5504=CARTESIAN_POINT('Origin',(0.,-0.166705,0.));
#5505=CARTESIAN_POINT('',(0.242834539687906,-0.04763,0.989696097314));
#5506=CARTESIAN_POINT('Origin',(0.,-0.04763,0.));
#5507=CARTESIAN_POINT('',(-0.242834539687907,-0.04763,0.989696097314));
#5508=CARTESIAN_POINT('Ctrl Pts',(0.242834539687906,-0.04763,0.989696097314));
#5509=CARTESIAN_POINT('Ctrl Pts',(0.24024064412003,-0.0609922781173483,
0.990332542620729));
#5510=CARTESIAN_POINT('Ctrl Pts',(0.236509675094874,-0.0742967091364492,
0.991238884025248));
#5511=CARTESIAN_POINT('Ctrl Pts',(0.221129100087819,-0.115492077056649,
0.994830026707808));
#5512=CARTESIAN_POINT('Ctrl Pts',(0.205111543747588,-0.141695629206859,
0.998375294985966));
#5513=CARTESIAN_POINT('Ctrl Pts',(0.169940289819232,-0.181890537957859,
1.00492400591205));
#5514=CARTESIAN_POINT('Ctrl Pts',(0.1465689792446,-0.201072148666545,1.00869718865384));
#5515=CARTESIAN_POINT('Ctrl Pts',(0.106909345252087,-0.223955109275652,
1.01358704779679));
#5516=CARTESIAN_POINT('Ctrl Pts',(0.0861971848975941,-0.232742381310829,
1.0156297872271));
#5517=CARTESIAN_POINT('Ctrl Pts',(0.0430711894098822,-0.244234834628584,
1.01837060663223));
#5518=CARTESIAN_POINT('Ctrl Pts',(0.0206568624125605,-0.246942143572133,
1.019052));
#5519=CARTESIAN_POINT('Ctrl Pts',(-0.0206568624125608,-0.246942143572133,
1.019052));
#5520=CARTESIAN_POINT('Ctrl Pts',(-0.0430711894098825,-0.244234834628584,
1.01837060663223));
#5521=CARTESIAN_POINT('Ctrl Pts',(-0.0861971848975943,-0.232742381310829,
1.0156297872271));
#5522=CARTESIAN_POINT('Ctrl Pts',(-0.106909345252088,-0.223955109275652,
1.01358704779679));
#5523=CARTESIAN_POINT('Ctrl Pts',(-0.1465689792446,-0.201072148666545,1.00869718865384));
#5524=CARTESIAN_POINT('Ctrl Pts',(-0.169940289819232,-0.181890537957859,
1.00492400591205));
#5525=CARTESIAN_POINT('Ctrl Pts',(-0.205111543747588,-0.141695629206859,
0.998375294985966));
#5526=CARTESIAN_POINT('Ctrl Pts',(-0.221129100087819,-0.115492077056649,
0.994830026707808));
#5527=CARTESIAN_POINT('Ctrl Pts',(-0.236509675094875,-0.0742967091364493,
0.991238884025248));
#5528=CARTESIAN_POINT('Ctrl Pts',(-0.24024064412003,-0.0609922781173483,
0.990332542620729));
#5529=CARTESIAN_POINT('Ctrl Pts',(-0.242834539687907,-0.04763,0.989696097314));
#5530=CARTESIAN_POINT('',(-0.528110872004959,-0.04763,0.871530771444223));
#5531=CARTESIAN_POINT('Origin',(0.,-0.04763,0.));
#5532=CARTESIAN_POINT('',(-0.871530771444223,-0.04763,0.528110872004958));
#5533=CARTESIAN_POINT('Ctrl Pts',(-0.528110872004958,-0.0476300000000001,
0.871530771444223));
#5534=CARTESIAN_POINT('Ctrl Pts',(-0.530395067942936,-0.0609922781173484,
0.87014664509073));
#5535=CARTESIAN_POINT('Ctrl Pts',(-0.533674141594226,-0.0742967091364493,
0.868149331745851));
#5536=CARTESIAN_POINT('Ctrl Pts',(-0.54708917182331,-0.115492077056649,
0.85981294420286));
#5537=CARTESIAN_POINT('Ctrl Pts',(-0.560922177770136,-0.141695629206859,
0.850993704737257));
#5538=CARTESIAN_POINT('Ctrl Pts',(-0.590422647829571,-0.181890537957859,
0.830754510485543));
#5539=CARTESIAN_POINT('Ctrl Pts',(-0.609616703125488,-0.201072148666545,
0.816896541396381));
#5540=CARTESIAN_POINT('Ctrl Pts',(-0.641117951819998,-0.223955109275652,
0.792310597819928));
#5541=CARTESIAN_POINT('Ctrl Pts',(-0.657208095763053,-0.232742381310829,
0.779109323683611));
#5542=CARTESIAN_POINT('Ctrl Pts',(-0.68964083160521,-0.244234834628584,
0.750552691816205));
#5543=CARTESIAN_POINT('Ctrl Pts',(-0.705971972091755,-0.246942143572133,
0.735185187071673));
#5544=CARTESIAN_POINT('Ctrl Pts',(-0.735185187071673,-0.246942143572133,
0.705971972091754));
#5545=CARTESIAN_POINT('Ctrl Pts',(-0.750552691816206,-0.244234834628584,
0.689640831605209));
#5546=CARTESIAN_POINT('Ctrl Pts',(-0.779109323683612,-0.232742381310829,
0.657208095763052));
#5547=CARTESIAN_POINT('Ctrl Pts',(-0.792310597819928,-0.223955109275652,
0.641117951819998));
#5548=CARTESIAN_POINT('Ctrl Pts',(-0.816896541396382,-0.201072148666545,
0.609616703125487));
#5549=CARTESIAN_POINT('Ctrl Pts',(-0.830754510485544,-0.181890537957858,
0.590422647829571));
#5550=CARTESIAN_POINT('Ctrl Pts',(-0.850993704737257,-0.141695629206858,
0.560922177770135));
#5551=CARTESIAN_POINT('Ctrl Pts',(-0.859812944202861,-0.115492077056649,
0.547089171823309));
#5552=CARTESIAN_POINT('Ctrl Pts',(-0.868149331745852,-0.0742967091364491,
0.533674141594226));
#5553=CARTESIAN_POINT('Ctrl Pts',(-0.870146645090731,-0.0609922781173483,
0.530395067942936));
#5554=CARTESIAN_POINT('Ctrl Pts',(-0.871530771444223,-0.04763,0.528110872004958));
#5555=CARTESIAN_POINT('',(-0.989696097314,-0.04763,0.242834539687906));
#5556=CARTESIAN_POINT('Origin',(0.,-0.04763,0.));
#5557=CARTESIAN_POINT('',(-1.019052,-0.246942143572133,1.248489836334E-16));
#5558=CARTESIAN_POINT('Ctrl Pts',(-0.989696097314,-0.04763,0.242834539687906));
#5559=CARTESIAN_POINT('Ctrl Pts',(-0.990332542620729,-0.0609922781173483,
0.24024064412003));
#5560=CARTESIAN_POINT('Ctrl Pts',(-0.991238884025248,-0.0742967091364492,
0.236509675094874));
#5561=CARTESIAN_POINT('Ctrl Pts',(-0.994830026707808,-0.115492077056649,
0.221129100087819));
#5562=CARTESIAN_POINT('Ctrl Pts',(-0.998375294985966,-0.141695629206859,
0.205111543747588));
#5563=CARTESIAN_POINT('Ctrl Pts',(-1.00492400591205,-0.181890537957859,
0.169940289819232));
#5564=CARTESIAN_POINT('Ctrl Pts',(-1.00869718865384,-0.201072148666545,
0.1465689792446));
#5565=CARTESIAN_POINT('Ctrl Pts',(-1.01358704779679,-0.223955109275652,
0.106909345252088));
#5566=CARTESIAN_POINT('Ctrl Pts',(-1.0156297872271,-0.232742381310829,0.0861971848975944));
#5567=CARTESIAN_POINT('Ctrl Pts',(-1.01837060663223,-0.244234834628584,
0.0430711894098825));
#5568=CARTESIAN_POINT('Ctrl Pts',(-1.019052,-0.246942143572133,0.0206568624125608));
#5569=CARTESIAN_POINT('Ctrl Pts',(-1.019052,-0.246942143572133,1.2490009027033E-16));
#5570=CARTESIAN_POINT('',(-1.019052,-0.28578,1.24797876996471E-16));
#5571=CARTESIAN_POINT('',(-1.019052,-0.166705,1.24797876996471E-16));
#5572=CARTESIAN_POINT('Origin',(0.,-0.28578,0.));
#5573=CARTESIAN_POINT('',(-0.989696097314,-0.04763,-0.242834539687906));
#5574=CARTESIAN_POINT('Ctrl Pts',(-1.019052,-0.246942143572133,1.2490009027033E-16));
#5575=CARTESIAN_POINT('Ctrl Pts',(-1.019052,-0.246942143572133,-0.0206568624125605));
#5576=CARTESIAN_POINT('Ctrl Pts',(-1.01837060663223,-0.244234834628584,
-0.0430711894098822));
#5577=CARTESIAN_POINT('Ctrl Pts',(-1.0156297872271,-0.232742381310829,-0.0861971848975941));
#5578=CARTESIAN_POINT('Ctrl Pts',(-1.01358704779679,-0.223955109275652,
-0.106909345252087));
#5579=CARTESIAN_POINT('Ctrl Pts',(-1.00869718865384,-0.201072148666546,
-0.1465689792446));
#5580=CARTESIAN_POINT('Ctrl Pts',(-1.00492400591205,-0.181890537957859,
-0.169940289819232));
#5581=CARTESIAN_POINT('Ctrl Pts',(-0.998375294985966,-0.141695629206859,
-0.205111543747588));
#5582=CARTESIAN_POINT('Ctrl Pts',(-0.994830026707808,-0.11549207705665,
-0.221129100087819));
#5583=CARTESIAN_POINT('Ctrl Pts',(-0.991238884025248,-0.0742967091364495,
-0.236509675094874));
#5584=CARTESIAN_POINT('Ctrl Pts',(-0.990332542620729,-0.0609922781173484,
-0.24024064412003));
#5585=CARTESIAN_POINT('Ctrl Pts',(-0.989696097314,-0.0476300000000001,-0.242834539687907));
#5586=CARTESIAN_POINT('',(-0.871530771444223,-0.04763,-0.528110872004958));
#5587=CARTESIAN_POINT('Origin',(0.,-0.04763,0.));
#5588=CARTESIAN_POINT('',(-0.528110872004958,-0.04763,-0.871530771444223));
#5589=CARTESIAN_POINT('Ctrl Pts',(-0.871530771444223,-0.0476300000000001,
-0.528110872004958));
#5590=CARTESIAN_POINT('Ctrl Pts',(-0.87014664509073,-0.0609922781173484,
-0.530395067942936));
#5591=CARTESIAN_POINT('Ctrl Pts',(-0.868149331745851,-0.0742967091364494,
-0.533674141594226));
#5592=CARTESIAN_POINT('Ctrl Pts',(-0.85981294420286,-0.115492077056649,
-0.54708917182331));
#5593=CARTESIAN_POINT('Ctrl Pts',(-0.850993704737257,-0.141695629206859,
-0.560922177770136));
#5594=CARTESIAN_POINT('Ctrl Pts',(-0.830754510485543,-0.181890537957859,
-0.590422647829571));
#5595=CARTESIAN_POINT('Ctrl Pts',(-0.816896541396381,-0.201072148666546,
-0.609616703125488));
#5596=CARTESIAN_POINT('Ctrl Pts',(-0.792310597819928,-0.223955109275652,
-0.641117951819999));
#5597=CARTESIAN_POINT('Ctrl Pts',(-0.779109323683611,-0.232742381310829,
-0.657208095763053));
#5598=CARTESIAN_POINT('Ctrl Pts',(-0.750552691816205,-0.244234834628584,
-0.68964083160521));
#5599=CARTESIAN_POINT('Ctrl Pts',(-0.735185187071673,-0.246942143572133,
-0.705971972091755));
#5600=CARTESIAN_POINT('Ctrl Pts',(-0.705971972091754,-0.246942143572133,
-0.735185187071673));
#5601=CARTESIAN_POINT('Ctrl Pts',(-0.68964083160521,-0.244234834628584,
-0.750552691816206));
#5602=CARTESIAN_POINT('Ctrl Pts',(-0.657208095763052,-0.232742381310829,
-0.779109323683612));
#5603=CARTESIAN_POINT('Ctrl Pts',(-0.641117951819998,-0.223955109275652,
-0.792310597819928));
#5604=CARTESIAN_POINT('Ctrl Pts',(-0.609616703125488,-0.201072148666545,
-0.816896541396381));
#5605=CARTESIAN_POINT('Ctrl Pts',(-0.590422647829571,-0.181890537957859,
-0.830754510485543));
#5606=CARTESIAN_POINT('Ctrl Pts',(-0.560922177770136,-0.141695629206859,
-0.850993704737257));
#5607=CARTESIAN_POINT('Ctrl Pts',(-0.54708917182331,-0.115492077056649,
-0.85981294420286));
#5608=CARTESIAN_POINT('Ctrl Pts',(-0.533674141594226,-0.0742967091364494,
-0.868149331745852));
#5609=CARTESIAN_POINT('Ctrl Pts',(-0.530395067942936,-0.0609922781173484,
-0.870146645090731));
#5610=CARTESIAN_POINT('Ctrl Pts',(-0.528110872004958,-0.0476300000000001,
-0.871530771444223));
#5611=CARTESIAN_POINT('',(-0.242834539687906,-0.04763,-0.989696097314));
#5612=CARTESIAN_POINT('Origin',(0.,-0.04763,0.));
#5613=CARTESIAN_POINT('',(0.242834539687906,-0.04763,-0.989696097314));
#5614=CARTESIAN_POINT('Ctrl Pts',(-0.242834539687907,-0.04763,-0.989696097314));
#5615=CARTESIAN_POINT('Ctrl Pts',(-0.24024064412003,-0.0609922781173483,
-0.990332542620729));
#5616=CARTESIAN_POINT('Ctrl Pts',(-0.236509675094874,-0.0742967091364493,
-0.991238884025248));
#5617=CARTESIAN_POINT('Ctrl Pts',(-0.221129100087819,-0.115492077056649,
-0.994830026707808));
#5618=CARTESIAN_POINT('Ctrl Pts',(-0.205111543747588,-0.141695629206859,
-0.998375294985966));
#5619=CARTESIAN_POINT('Ctrl Pts',(-0.169940289819232,-0.181890537957859,
-1.00492400591205));
#5620=CARTESIAN_POINT('Ctrl Pts',(-0.1465689792446,-0.201072148666545,-1.00869718865384));
#5621=CARTESIAN_POINT('Ctrl Pts',(-0.106909345252087,-0.223955109275652,
-1.01358704779679));
#5622=CARTESIAN_POINT('Ctrl Pts',(-0.0861971848975942,-0.232742381310829,
-1.0156297872271));
#5623=CARTESIAN_POINT('Ctrl Pts',(-0.0430711894098823,-0.244234834628584,
-1.01837060663223));
#5624=CARTESIAN_POINT('Ctrl Pts',(-0.0206568624125606,-0.246942143572133,
-1.019052));
#5625=CARTESIAN_POINT('Ctrl Pts',(0.0206568624125607,-0.246942143572133,
-1.019052));
#5626=CARTESIAN_POINT('Ctrl Pts',(0.0430711894098824,-0.244234834628584,
-1.01837060663223));
#5627=CARTESIAN_POINT('Ctrl Pts',(0.0861971848975943,-0.232742381310829,
-1.0156297872271));
#5628=CARTESIAN_POINT('Ctrl Pts',(0.106909345252088,-0.223955109275652,
-1.01358704779679));
#5629=CARTESIAN_POINT('Ctrl Pts',(0.1465689792446,-0.201072148666545,-1.00869718865384));
#5630=CARTESIAN_POINT('Ctrl Pts',(0.169940289819232,-0.181890537957859,
-1.00492400591205));
#5631=CARTESIAN_POINT('Ctrl Pts',(0.205111543747588,-0.141695629206859,
-0.998375294985966));
#5632=CARTESIAN_POINT('Ctrl Pts',(0.221129100087819,-0.115492077056649,
-0.994830026707808));
#5633=CARTESIAN_POINT('Ctrl Pts',(0.236509675094874,-0.0742967091364493,
-0.991238884025248));
#5634=CARTESIAN_POINT('Ctrl Pts',(0.24024064412003,-0.0609922781173484,
-0.990332542620729));
#5635=CARTESIAN_POINT('Ctrl Pts',(0.242834539687907,-0.04763,-0.989696097314));
#5636=CARTESIAN_POINT('',(0.528110872004958,-0.04763,-0.871530771444223));
#5637=CARTESIAN_POINT('Origin',(0.,-0.04763,0.));
#5638=CARTESIAN_POINT('',(0.871530771444223,-0.04763,-0.528110872004958));
#5639=CARTESIAN_POINT('Ctrl Pts',(0.528110872004958,-0.0476300000000001,
-0.871530771444223));
#5640=CARTESIAN_POINT('Ctrl Pts',(0.530395067942936,-0.0609922781173484,
-0.870146645090731));
#5641=CARTESIAN_POINT('Ctrl Pts',(0.533674141594226,-0.0742967091364493,
-0.868149331745851));
#5642=CARTESIAN_POINT('Ctrl Pts',(0.54708917182331,-0.115492077056649,-0.85981294420286));
#5643=CARTESIAN_POINT('Ctrl Pts',(0.560922177770136,-0.141695629206859,
-0.850993704737257));
#5644=CARTESIAN_POINT('Ctrl Pts',(0.590422647829571,-0.181890537957859,
-0.830754510485543));
#5645=CARTESIAN_POINT('Ctrl Pts',(0.609616703125488,-0.201072148666545,
-0.816896541396381));
#5646=CARTESIAN_POINT('Ctrl Pts',(0.641117951819998,-0.223955109275652,
-0.792310597819928));
#5647=CARTESIAN_POINT('Ctrl Pts',(0.657208095763053,-0.232742381310829,
-0.779109323683612));
#5648=CARTESIAN_POINT('Ctrl Pts',(0.68964083160521,-0.244234834628584,-0.750552691816206));
#5649=CARTESIAN_POINT('Ctrl Pts',(0.705971972091755,-0.246942143572133,
-0.735185187071673));
#5650=CARTESIAN_POINT('Ctrl Pts',(0.735185187071673,-0.246942143572133,
-0.705971972091754));
#5651=CARTESIAN_POINT('Ctrl Pts',(0.750552691816206,-0.244234834628584,
-0.68964083160521));
#5652=CARTESIAN_POINT('Ctrl Pts',(0.779109323683612,-0.232742381310829,
-0.657208095763053));
#5653=CARTESIAN_POINT('Ctrl Pts',(0.792310597819928,-0.223955109275652,
-0.641117951819998));
#5654=CARTESIAN_POINT('Ctrl Pts',(0.816896541396381,-0.201072148666545,
-0.609616703125488));
#5655=CARTESIAN_POINT('Ctrl Pts',(0.830754510485543,-0.181890537957859,
-0.590422647829571));
#5656=CARTESIAN_POINT('Ctrl Pts',(0.850993704737257,-0.141695629206859,
-0.560922177770136));
#5657=CARTESIAN_POINT('Ctrl Pts',(0.85981294420286,-0.115492077056649,-0.54708917182331));
#5658=CARTESIAN_POINT('Ctrl Pts',(0.868149331745851,-0.0742967091364493,
-0.533674141594226));
#5659=CARTESIAN_POINT('Ctrl Pts',(0.870146645090731,-0.0609922781173484,
-0.530395067942936));
#5660=CARTESIAN_POINT('Ctrl Pts',(0.871530771444223,-0.0476300000000001,
-0.528110872004958));
#5661=CARTESIAN_POINT('',(0.989696097314,-0.04763,-0.242834539687906));
#5662=CARTESIAN_POINT('Origin',(0.,-0.04763,0.));
#5663=CARTESIAN_POINT('',(0.989696097314,-0.04763,0.242834539687906));
#5664=CARTESIAN_POINT('Ctrl Pts',(0.989696097314,-0.04763,-0.242834539687907));
#5665=CARTESIAN_POINT('Ctrl Pts',(0.990332542620729,-0.0609922781173483,
-0.24024064412003));
#5666=CARTESIAN_POINT('Ctrl Pts',(0.991238884025248,-0.0742967091364493,
-0.236509675094874));
#5667=CARTESIAN_POINT('Ctrl Pts',(0.994830026707808,-0.115492077056649,
-0.221129100087819));
#5668=CARTESIAN_POINT('Ctrl Pts',(0.998375294985966,-0.141695629206859,
-0.205111543747588));
#5669=CARTESIAN_POINT('Ctrl Pts',(1.00492400591205,-0.181890537957859,-0.169940289819232));
#5670=CARTESIAN_POINT('Ctrl Pts',(1.00869718865384,-0.201072148666545,-0.1465689792446));
#5671=CARTESIAN_POINT('Ctrl Pts',(1.01358704779679,-0.223955109275652,-0.106909345252087));
#5672=CARTESIAN_POINT('Ctrl Pts',(1.0156297872271,-0.232742381310829,-0.0861971848975942));
#5673=CARTESIAN_POINT('Ctrl Pts',(1.01837060663223,-0.244234834628584,-0.0430711894098823));
#5674=CARTESIAN_POINT('Ctrl Pts',(1.019052,-0.246942143572133,-0.0206568624125607));
#5675=CARTESIAN_POINT('Ctrl Pts',(1.019052,-0.246942143572133,0.0206568624125607));
#5676=CARTESIAN_POINT('Ctrl Pts',(1.01837060663223,-0.244234834628584,0.0430711894098823));
#5677=CARTESIAN_POINT('Ctrl Pts',(1.0156297872271,-0.232742381310829,0.0861971848975942));
#5678=CARTESIAN_POINT('Ctrl Pts',(1.01358704779679,-0.223955109275652,0.106909345252087));
#5679=CARTESIAN_POINT('Ctrl Pts',(1.00869718865384,-0.201072148666545,0.1465689792446));
#5680=CARTESIAN_POINT('Ctrl Pts',(1.00492400591205,-0.181890537957859,0.169940289819232));
#5681=CARTESIAN_POINT('Ctrl Pts',(0.998375294985966,-0.141695629206859,
0.205111543747588));
#5682=CARTESIAN_POINT('Ctrl Pts',(0.994830026707808,-0.115492077056649,
0.221129100087819));
#5683=CARTESIAN_POINT('Ctrl Pts',(0.991238884025248,-0.0742967091364492,
0.236509675094874));
#5684=CARTESIAN_POINT('Ctrl Pts',(0.990332542620729,-0.0609922781173483,
0.24024064412003));
#5685=CARTESIAN_POINT('Ctrl Pts',(0.989696097314,-0.04763,0.242834539687907));
#5686=CARTESIAN_POINT('Origin',(0.,-0.04763,0.));
#5687=CARTESIAN_POINT('Origin',(0.,-0.04763,0.));
#5688=CARTESIAN_POINT('',(0.238183666596899,-0.04763,0.951592097314));
#5689=CARTESIAN_POINT('Origin',(0.,-0.04763,0.));
#5690=CARTESIAN_POINT('Origin',(-1.94289029309402E-16,-0.04763,1.));
#5691=CARTESIAN_POINT('Origin',(-1.94289029309402E-16,0.,1.));
#5692=CARTESIAN_POINT('',(-0.2381836665969,-0.04763,0.951592097314));
#5693=CARTESIAN_POINT('Ctrl Pts',(-0.238183666596899,-0.0476299999999999,
0.951592097314));
#5694=CARTESIAN_POINT('Ctrl Pts',(-0.233157223576062,-0.0740444353928835,
0.952850216871763));
#5695=CARTESIAN_POINT('Ctrl Pts',(-0.223801617934946,-0.0999305678883309,
0.955173119738174));
#5696=CARTESIAN_POINT('Ctrl Pts',(-0.199966927975188,-0.142345102874864,
0.960411259488514));
#5697=CARTESIAN_POINT('Ctrl Pts',(-0.1868781821531,-0.159766064500479,0.963103647174702));
#5698=CARTESIAN_POINT('Ctrl Pts',(-0.15681442133453,-0.190326085855194,
0.968453058988463));
#5699=CARTESIAN_POINT('Ctrl Pts',(-0.139836317888043,-0.203463743702801,
0.971100730005489));
#5700=CARTESIAN_POINT('Ctrl Pts',(-0.104422493053067,-0.224161999508995,
0.975530745318961));
#5701=CARTESIAN_POINT('Ctrl Pts',(-0.0842175114474176,-0.232861760990032,
0.977553872336861));
#5702=CARTESIAN_POINT('Ctrl Pts',(-0.0421062857595701,-0.244251601209411,
0.980270995488453));
#5703=CARTESIAN_POINT('Ctrl Pts',(-0.0201990724523197,-0.246942143572133,
0.980948));
#5704=CARTESIAN_POINT('Ctrl Pts',(0.020199072452319,-0.246942143572133,
0.980948));
#5705=CARTESIAN_POINT('Ctrl Pts',(0.0421062857595694,-0.244251601209411,
0.980270995488454));
#5706=CARTESIAN_POINT('Ctrl Pts',(0.0842175114474169,-0.232861760990032,
0.977553872336861));
#5707=CARTESIAN_POINT('Ctrl Pts',(0.104422493053067,-0.224161999508995,
0.975530745318961));
#5708=CARTESIAN_POINT('Ctrl Pts',(0.139836317888042,-0.203463743702801,
0.971100730005489));
#5709=CARTESIAN_POINT('Ctrl Pts',(0.15681442133453,-0.190326085855194,0.968453058988463));
#5710=CARTESIAN_POINT('Ctrl Pts',(0.1868781821531,-0.15976606450048,0.963103647174702));
#5711=CARTESIAN_POINT('Ctrl Pts',(0.199966927975188,-0.142345102874864,
0.960411259488514));
#5712=CARTESIAN_POINT('Ctrl Pts',(0.223801617934945,-0.0999305678883309,
0.955173119738174));
#5713=CARTESIAN_POINT('Ctrl Pts',(0.233157223576061,-0.0740444353928835,
0.952850216871763));
#5714=CARTESIAN_POINT('Ctrl Pts',(0.238183666596899,-0.0476299999999999,
0.951592097314));
#5715=CARTESIAN_POINT('Origin',(-1.94289029309402E-16,-0.04763,1.));
#5716=CARTESIAN_POINT('Origin',(0.,-0.04763,0.));
#5717=CARTESIAN_POINT('',(-0.504455939115715,-0.04763,0.841298510752802));
#5718=CARTESIAN_POINT('Origin',(0.,-0.04763,0.));
#5719=CARTESIAN_POINT('Origin',(-0.707106781186548,-0.04763,0.707106781186547));
#5720=CARTESIAN_POINT('Origin',(-0.707106781186548,0.,0.707106781186547));
#5721=CARTESIAN_POINT('',(-0.841298510752802,-0.04763,0.504455939115715));
#5722=CARTESIAN_POINT('Ctrl Pts',(-0.841298510752802,-0.04763,0.504455939115715));
#5723=CARTESIAN_POINT('Ctrl Pts',(-0.838633903678357,-0.0740444353928835,
0.508899795931835));
#5724=CARTESIAN_POINT('Ctrl Pts',(-0.833661031856294,-0.0999305678883309,
0.517157748491652));
#5725=CARTESIAN_POINT('Ctrl Pts',(-0.820511285096538,-0.142345102874864,
0.537715343527944));
#5726=CARTESIAN_POINT('Ctrl Pts',(-0.813159949759,-0.159766064500479,0.548874290046456));
#5727=CARTESIAN_POINT('Ctrl Pts',(-0.795684265985089,-0.190326085855194,
0.573915184558107));
#5728=CARTESIAN_POINT('Ctrl Pts',(-0.78555112003688,-0.203463743702801,
0.587792702767295));
#5729=CARTESIAN_POINT('Ctrl Pts',(-0.763642258217233,-0.224161999508995,
0.615966552324775));
#5730=CARTESIAN_POINT('Ctrl Pts',(-0.750785745543687,-0.232861760990032,
0.631684198665438));
#5731=CARTESIAN_POINT('Ctrl Pts',(-0.722929908501543,-0.244251601209411,
0.663382628119203));
#5732=CARTESIAN_POINT('Ctrl Pts',(-0.707917883896095,-0.246942143572133,
0.679352081686668));
#5733=CARTESIAN_POINT('Ctrl Pts',(-0.679352081686668,-0.246942143572133,
0.707917883896095));
#5734=CARTESIAN_POINT('Ctrl Pts',(-0.663382628119203,-0.244251601209411,
0.722929908501544));
#5735=CARTESIAN_POINT('Ctrl Pts',(-0.631684198665438,-0.232861760990031,
0.750785745543687));
#5736=CARTESIAN_POINT('Ctrl Pts',(-0.615966552324775,-0.224161999508995,
0.763642258217233));
#5737=CARTESIAN_POINT('Ctrl Pts',(-0.587792702767295,-0.203463743702801,
0.78555112003688));
#5738=CARTESIAN_POINT('Ctrl Pts',(-0.573915184558107,-0.190326085855194,
0.795684265985088));
#5739=CARTESIAN_POINT('Ctrl Pts',(-0.548874290046456,-0.159766064500479,
0.813159949759));
#5740=CARTESIAN_POINT('Ctrl Pts',(-0.537715343527944,-0.142345102874864,
0.820511285096538));
#5741=CARTESIAN_POINT('Ctrl Pts',(-0.517157748491652,-0.0999305678883309,
0.833661031856294));
#5742=CARTESIAN_POINT('Ctrl Pts',(-0.508899795931835,-0.0740444353928835,
0.838633903678357));
#5743=CARTESIAN_POINT('Ctrl Pts',(-0.504455939115716,-0.04763,0.841298510752801));
#5744=CARTESIAN_POINT('Origin',(-0.707106781186548,-0.04763,0.707106781186547));
#5745=CARTESIAN_POINT('Origin',(0.,-0.04763,0.));
#5746=CARTESIAN_POINT('',(-0.951592097314,-0.04763,0.238183666596899));
#5747=CARTESIAN_POINT('Origin',(0.,-0.04763,0.));
#5748=CARTESIAN_POINT('Origin',(-1.,-0.04763,-1.11022302462516E-16));
#5749=CARTESIAN_POINT('Origin',(-1.,0.,-1.11022302462516E-16));
#5750=CARTESIAN_POINT('',(-0.951592097314,-0.04763,-0.2381836665969));
#5751=CARTESIAN_POINT('',(-0.980948,-0.246942143572133,1.08514323328844E-18));
#5752=CARTESIAN_POINT('Ctrl Pts',(-0.951592097314,-0.04763,-0.238183666596899));
#5753=CARTESIAN_POINT('Ctrl Pts',(-0.952850216871763,-0.0740444353928835,
-0.233157223576062));
#5754=CARTESIAN_POINT('Ctrl Pts',(-0.955173119738174,-0.0999305678883309,
-0.223801617934946));
#5755=CARTESIAN_POINT('Ctrl Pts',(-0.960411259488514,-0.142345102874864,
-0.199966927975188));
#5756=CARTESIAN_POINT('Ctrl Pts',(-0.963103647174702,-0.159766064500479,
-0.1868781821531));
#5757=CARTESIAN_POINT('Ctrl Pts',(-0.968453058988463,-0.190326085855194,
-0.15681442133453));
#5758=CARTESIAN_POINT('Ctrl Pts',(-0.971100730005489,-0.203463743702801,
-0.139836317888043));
#5759=CARTESIAN_POINT('Ctrl Pts',(-0.975530745318961,-0.224161999508995,
-0.104422493053067));
#5760=CARTESIAN_POINT('Ctrl Pts',(-0.977553872336861,-0.232861760990032,
-0.0842175114474175));
#5761=CARTESIAN_POINT('Ctrl Pts',(-0.980270995488453,-0.244251601209411,
-0.0421062857595699));
#5762=CARTESIAN_POINT('Ctrl Pts',(-0.980948,-0.246942143572133,-0.0201990724523195));
#5763=CARTESIAN_POINT('Ctrl Pts',(-0.980948,-0.246942143572133,-1.17961196366423E-16));
#5764=CARTESIAN_POINT('Origin',(-1.,-0.04763,-1.11022302462516E-16));
#5765=CARTESIAN_POINT('Ctrl Pts',(-0.980948,-0.246942143572133,-1.17961196366423E-16));
#5766=CARTESIAN_POINT('Ctrl Pts',(-0.980948,-0.246942143572133,0.0201990724523192));
#5767=CARTESIAN_POINT('Ctrl Pts',(-0.980270995488453,-0.244251601209411,
0.0421062857595695));
#5768=CARTESIAN_POINT('Ctrl Pts',(-0.977553872336861,-0.232861760990032,
0.0842175114474169));
#5769=CARTESIAN_POINT('Ctrl Pts',(-0.975530745318961,-0.224161999508995,
0.104422493053066));
#5770=CARTESIAN_POINT('Ctrl Pts',(-0.971100730005489,-0.203463743702801,
0.139836317888042));
#5771=CARTESIAN_POINT('Ctrl Pts',(-0.968453058988463,-0.190326085855194,
0.15681442133453));
#5772=CARTESIAN_POINT('Ctrl Pts',(-0.963103647174702,-0.15976606450048,
0.1868781821531));
#5773=CARTESIAN_POINT('Ctrl Pts',(-0.960411259488514,-0.142345102874864,
0.199966927975188));
#5774=CARTESIAN_POINT('Ctrl Pts',(-0.955173119738174,-0.099930567888331,
0.223801617934945));
#5775=CARTESIAN_POINT('Ctrl Pts',(-0.952850216871763,-0.0740444353928835,
0.233157223576061));
#5776=CARTESIAN_POINT('Ctrl Pts',(-0.951592097314,-0.04763,0.238183666596899));
#5777=CARTESIAN_POINT('Origin',(0.,-0.04763,0.));
#5778=CARTESIAN_POINT('',(-0.841298510752802,-0.04763,-0.504455939115715));
#5779=CARTESIAN_POINT('Origin',(0.,-0.04763,0.));
#5780=CARTESIAN_POINT('Origin',(-0.707106781186547,-0.04763,-0.707106781186548));
#5781=CARTESIAN_POINT('Origin',(-0.707106781186547,0.,-0.707106781186548));
#5782=CARTESIAN_POINT('',(-0.504455939115715,-0.04763,-0.841298510752802));
#5783=CARTESIAN_POINT('Ctrl Pts',(-0.504455939115715,-0.04763,-0.841298510752802));
#5784=CARTESIAN_POINT('Ctrl Pts',(-0.508899795931835,-0.0740444353928835,
-0.838633903678357));
#5785=CARTESIAN_POINT('Ctrl Pts',(-0.517157748491652,-0.0999305678883309,
-0.833661031856294));
#5786=CARTESIAN_POINT('Ctrl Pts',(-0.537715343527944,-0.142345102874864,
-0.820511285096538));
#5787=CARTESIAN_POINT('Ctrl Pts',(-0.548874290046456,-0.159766064500479,
-0.813159949759));
#5788=CARTESIAN_POINT('Ctrl Pts',(-0.573915184558107,-0.190326085855194,
-0.795684265985089));
#5789=CARTESIAN_POINT('Ctrl Pts',(-0.587792702767295,-0.203463743702801,
-0.78555112003688));
#5790=CARTESIAN_POINT('Ctrl Pts',(-0.615966552324775,-0.224161999508995,
-0.763642258217233));
#5791=CARTESIAN_POINT('Ctrl Pts',(-0.631684198665438,-0.232861760990032,
-0.750785745543687));
#5792=CARTESIAN_POINT('Ctrl Pts',(-0.663382628119203,-0.244251601209411,
-0.722929908501543));
#5793=CARTESIAN_POINT('Ctrl Pts',(-0.679352081686668,-0.246942143572133,
-0.707917883896095));
#5794=CARTESIAN_POINT('Ctrl Pts',(-0.707917883896095,-0.246942143572133,
-0.679352081686668));
#5795=CARTESIAN_POINT('Ctrl Pts',(-0.722929908501543,-0.244251601209411,
-0.663382628119203));
#5796=CARTESIAN_POINT('Ctrl Pts',(-0.750785745543687,-0.232861760990032,
-0.631684198665439));
#5797=CARTESIAN_POINT('Ctrl Pts',(-0.763642258217232,-0.224161999508995,
-0.615966552324775));
#5798=CARTESIAN_POINT('Ctrl Pts',(-0.78555112003688,-0.203463743702801,
-0.587792702767295));
#5799=CARTESIAN_POINT('Ctrl Pts',(-0.795684265985088,-0.190326085855194,
-0.573915184558107));
#5800=CARTESIAN_POINT('Ctrl Pts',(-0.813159949759,-0.15976606450048,-0.548874290046456));
#5801=CARTESIAN_POINT('Ctrl Pts',(-0.820511285096538,-0.142345102874864,
-0.537715343527944));
#5802=CARTESIAN_POINT('Ctrl Pts',(-0.833661031856294,-0.0999305678883311,
-0.517157748491652));
#5803=CARTESIAN_POINT('Ctrl Pts',(-0.838633903678357,-0.0740444353928836,
-0.508899795931835));
#5804=CARTESIAN_POINT('Ctrl Pts',(-0.841298510752801,-0.04763,-0.504455939115715));
#5805=CARTESIAN_POINT('Origin',(-0.707106781186547,-0.04763,-0.707106781186548));
#5806=CARTESIAN_POINT('Origin',(0.,-0.04763,0.));
#5807=CARTESIAN_POINT('',(-0.238183666596899,-0.04763,-0.951592097314));
#5808=CARTESIAN_POINT('Origin',(0.,-0.04763,0.));
#5809=CARTESIAN_POINT('Origin',(5.55111512312578E-17,-0.04763,-1.));
#5810=CARTESIAN_POINT('Origin',(5.55111512312578E-17,0.,-1.));
#5811=CARTESIAN_POINT('',(0.238183666596899,-0.04763,-0.951592097314));
#5812=CARTESIAN_POINT('Ctrl Pts',(0.238183666596899,-0.04763,-0.951592097314));
#5813=CARTESIAN_POINT('Ctrl Pts',(0.233157223576062,-0.0740444353928835,
-0.952850216871763));
#5814=CARTESIAN_POINT('Ctrl Pts',(0.223801617934946,-0.099930567888331,
-0.955173119738174));
#5815=CARTESIAN_POINT('Ctrl Pts',(0.199966927975188,-0.142345102874864,
-0.960411259488514));
#5816=CARTESIAN_POINT('Ctrl Pts',(0.1868781821531,-0.15976606450048,-0.963103647174702));
#5817=CARTESIAN_POINT('Ctrl Pts',(0.15681442133453,-0.190326085855194,-0.968453058988463));
#5818=CARTESIAN_POINT('Ctrl Pts',(0.139836317888042,-0.203463743702801,
-0.971100730005489));
#5819=CARTESIAN_POINT('Ctrl Pts',(0.104422493053067,-0.224161999508995,
-0.975530745318961));
#5820=CARTESIAN_POINT('Ctrl Pts',(0.0842175114474173,-0.232861760990032,
-0.977553872336861));
#5821=CARTESIAN_POINT('Ctrl Pts',(0.0421062857595698,-0.244251601209411,
-0.980270995488453));
#5822=CARTESIAN_POINT('Ctrl Pts',(0.0201990724523194,-0.246942143572133,
-0.980948));
#5823=CARTESIAN_POINT('Ctrl Pts',(-0.0201990724523193,-0.246942143572133,
-0.980948));
#5824=CARTESIAN_POINT('Ctrl Pts',(-0.0421062857595697,-0.244251601209411,
-0.980270995488453));
#5825=CARTESIAN_POINT('Ctrl Pts',(-0.0842175114474171,-0.232861760990032,
-0.977553872336861));
#5826=CARTESIAN_POINT('Ctrl Pts',(-0.104422493053067,-0.224161999508995,
-0.975530745318961));
#5827=CARTESIAN_POINT('Ctrl Pts',(-0.139836317888042,-0.203463743702801,
-0.971100730005489));
#5828=CARTESIAN_POINT('Ctrl Pts',(-0.15681442133453,-0.190326085855194,
-0.968453058988463));
#5829=CARTESIAN_POINT('Ctrl Pts',(-0.1868781821531,-0.15976606450048,-0.963103647174702));
#5830=CARTESIAN_POINT('Ctrl Pts',(-0.199966927975188,-0.142345102874864,
-0.960411259488514));
#5831=CARTESIAN_POINT('Ctrl Pts',(-0.223801617934945,-0.099930567888331,
-0.955173119738174));
#5832=CARTESIAN_POINT('Ctrl Pts',(-0.233157223576062,-0.0740444353928835,
-0.952850216871763));
#5833=CARTESIAN_POINT('Ctrl Pts',(-0.238183666596899,-0.0476299999999999,
-0.951592097314));
#5834=CARTESIAN_POINT('Origin',(5.55111512312578E-17,-0.04763,-1.));
#5835=CARTESIAN_POINT('Origin',(0.,-0.04763,0.));
#5836=CARTESIAN_POINT('',(0.504455939115715,-0.04763,-0.841298510752802));
#5837=CARTESIAN_POINT('Origin',(0.,-0.04763,0.));
#5838=CARTESIAN_POINT('Origin',(0.707106781186548,-0.04763,-0.707106781186547));
#5839=CARTESIAN_POINT('Origin',(0.707106781186548,0.,-0.707106781186547));
#5840=CARTESIAN_POINT('',(0.841298510752802,-0.04763,-0.504455939115715));
#5841=CARTESIAN_POINT('Ctrl Pts',(0.841298510752802,-0.04763,-0.504455939115715));
#5842=CARTESIAN_POINT('Ctrl Pts',(0.838633903678357,-0.0740444353928835,
-0.508899795931835));
#5843=CARTESIAN_POINT('Ctrl Pts',(0.833661031856294,-0.0999305678883309,
-0.517157748491652));
#5844=CARTESIAN_POINT('Ctrl Pts',(0.820511285096538,-0.142345102874864,
-0.537715343527944));
#5845=CARTESIAN_POINT('Ctrl Pts',(0.813159949759,-0.159766064500479,-0.548874290046456));
#5846=CARTESIAN_POINT('Ctrl Pts',(0.795684265985088,-0.190326085855194,
-0.573915184558107));
#5847=CARTESIAN_POINT('Ctrl Pts',(0.78555112003688,-0.203463743702801,-0.587792702767295));
#5848=CARTESIAN_POINT('Ctrl Pts',(0.763642258217233,-0.224161999508995,
-0.615966552324775));
#5849=CARTESIAN_POINT('Ctrl Pts',(0.750785745543687,-0.232861760990032,
-0.631684198665438));
#5850=CARTESIAN_POINT('Ctrl Pts',(0.722929908501543,-0.244251601209411,
-0.663382628119203));
#5851=CARTESIAN_POINT('Ctrl Pts',(0.707917883896095,-0.246942143572133,
-0.679352081686668));
#5852=CARTESIAN_POINT('Ctrl Pts',(0.679352081686668,-0.246942143572133,
-0.707917883896095));
#5853=CARTESIAN_POINT('Ctrl Pts',(0.663382628119203,-0.244251601209411,
-0.722929908501543));
#5854=CARTESIAN_POINT('Ctrl Pts',(0.631684198665438,-0.232861760990032,
-0.750785745543687));
#5855=CARTESIAN_POINT('Ctrl Pts',(0.615966552324775,-0.224161999508995,
-0.763642258217232));
#5856=CARTESIAN_POINT('Ctrl Pts',(0.587792702767295,-0.203463743702801,
-0.78555112003688));
#5857=CARTESIAN_POINT('Ctrl Pts',(0.573915184558107,-0.190326085855194,
-0.795684265985088));
#5858=CARTESIAN_POINT('Ctrl Pts',(0.548874290046456,-0.159766064500479,
-0.813159949759));
#5859=CARTESIAN_POINT('Ctrl Pts',(0.537715343527944,-0.142345102874864,
-0.820511285096538));
#5860=CARTESIAN_POINT('Ctrl Pts',(0.517157748491652,-0.099930567888331,
-0.833661031856294));
#5861=CARTESIAN_POINT('Ctrl Pts',(0.508899795931835,-0.0740444353928835,
-0.838633903678357));
#5862=CARTESIAN_POINT('Ctrl Pts',(0.504455939115715,-0.04763,-0.841298510752801));
#5863=CARTESIAN_POINT('Origin',(0.707106781186548,-0.04763,-0.707106781186547));
#5864=CARTESIAN_POINT('Origin',(0.,-0.166705,0.));
#5865=CARTESIAN_POINT('',(-0.980948,-0.28578,1.20131482833E-16));
#5866=CARTESIAN_POINT('Origin',(0.,-0.28578,0.));
#5867=CARTESIAN_POINT('',(-0.980948,-0.166705,1.20131482833E-16));
#5868=CARTESIAN_POINT('',(0.951592097314,-0.04763,0.238183666596899));
#5869=CARTESIAN_POINT('Origin',(0.,-0.04763,0.));
#5870=CARTESIAN_POINT('',(0.951592097314,-0.04763,-0.238183666596899));
#5871=CARTESIAN_POINT('Ctrl Pts',(0.951592097314,-0.04763,0.238183666596899));
#5872=CARTESIAN_POINT('Ctrl Pts',(0.952850216871763,-0.0740444353928835,
0.233157223576062));
#5873=CARTESIAN_POINT('Ctrl Pts',(0.955173119738174,-0.099930567888331,
0.223801617934945));
#5874=CARTESIAN_POINT('Ctrl Pts',(0.960411259488514,-0.142345102874864,
0.199966927975188));
#5875=CARTESIAN_POINT('Ctrl Pts',(0.963103647174702,-0.15976606450048,0.1868781821531));
#5876=CARTESIAN_POINT('Ctrl Pts',(0.968453058988463,-0.190326085855194,
0.15681442133453));
#5877=CARTESIAN_POINT('Ctrl Pts',(0.971100730005489,-0.203463743702801,
0.139836317888042));
#5878=CARTESIAN_POINT('Ctrl Pts',(0.975530745318961,-0.224161999508995,
0.104422493053067));
#5879=CARTESIAN_POINT('Ctrl Pts',(0.977553872336861,-0.232861760990032,
0.0842175114474172));
#5880=CARTESIAN_POINT('Ctrl Pts',(0.980270995488453,-0.244251601209411,
0.0421062857595697));
#5881=CARTESIAN_POINT('Ctrl Pts',(0.980948,-0.246942143572133,0.0201990724523194));
#5882=CARTESIAN_POINT('Ctrl Pts',(0.980948,-0.246942143572133,-0.0201990724523194));
#5883=CARTESIAN_POINT('Ctrl Pts',(0.980270995488453,-0.244251601209411,
-0.0421062857595697));
#5884=CARTESIAN_POINT('Ctrl Pts',(0.977553872336861,-0.232861760990032,
-0.0842175114474172));
#5885=CARTESIAN_POINT('Ctrl Pts',(0.975530745318961,-0.224161999508995,
-0.104422493053067));
#5886=CARTESIAN_POINT('Ctrl Pts',(0.971100730005489,-0.203463743702801,
-0.139836317888042));
#5887=CARTESIAN_POINT('Ctrl Pts',(0.968453058988463,-0.190326085855194,
-0.15681442133453));
#5888=CARTESIAN_POINT('Ctrl Pts',(0.963103647174702,-0.15976606450048,-0.1868781821531));
#5889=CARTESIAN_POINT('Ctrl Pts',(0.960411259488514,-0.142345102874864,
-0.199966927975188));
#5890=CARTESIAN_POINT('Ctrl Pts',(0.955173119738174,-0.099930567888331,
-0.223801617934945));
#5891=CARTESIAN_POINT('Ctrl Pts',(0.952850216871763,-0.0740444353928835,
-0.233157223576062));
#5892=CARTESIAN_POINT('Ctrl Pts',(0.951592097314,-0.0476299999999999,-0.238183666596899));
#5893=CARTESIAN_POINT('Origin',(0.,-0.04763,0.));
#5894=CARTESIAN_POINT('Origin',(0.,-0.04763,0.));
#5895=CARTESIAN_POINT('Origin',(1.,-0.04763,0.));
#5896=CARTESIAN_POINT('Origin',(1.,0.,0.));
#5897=CARTESIAN_POINT('Origin',(1.,-0.04763,0.));
#5898=CARTESIAN_POINT('Origin',(0.,-0.28578,0.));
#5899=CARTESIAN_POINT('Origin',(0.,-0.04763,0.));
#6207=UNCERTAINTY_MEASURE_WITH_UNIT(LENGTH_MEASURE(0.001),#6242,
'DISTANCE_ACCURACY_VALUE',
'Maximum model space distance between geometric entities at asserted c
onnectivities');
#6215=UNCERTAINTY_MEASURE_WITH_UNIT(LENGTH_MEASURE(0.001),#6242,
'DISTANCE_ACCURACY_VALUE',
'Maximum model space distance between geometric entities at asserted c
onnectivities');
#6233=(
GEOMETRIC_REPRESENTATION_CONTEXT(3)
GLOBAL_UNCERTAINTY_ASSIGNED_CONTEXT((#6207))
GLOBAL_UNIT_ASSIGNED_CONTEXT((#6242,#6244,#6245))
REPRESENTATION_CONTEXT('','3D')
);
#6241=(
GEOMETRIC_REPRESENTATION_CONTEXT(3)
GLOBAL_UNCERTAINTY_ASSIGNED_CONTEXT((#6215))
GLOBAL_UNIT_ASSIGNED_CONTEXT((#6242,#6244,#6245))
REPRESENTATION_CONTEXT('','3D')
);
#6242=(
LENGTH_UNIT()
NAMED_UNIT(*)
SI_UNIT(.CENTI.,.METRE.)
);
#6244=(
NAMED_UNIT(*)
PLANE_ANGLE_UNIT()
SI_UNIT($,.RADIAN.)
);
#6245=(
NAMED_UNIT(*)
SI_UNIT($,.STERADIAN.)
SOLID_ANGLE_UNIT()
);
#6263=SHAPE_DEFINITION_REPRESENTATION(#6288,#6357);
#6288=PRODUCT_DEFINITION_SHAPE('',$,#6383);
#6357=SHAPE_REPRESENTATION('',(#3664),#6233);
#6365=PRODUCT_DEFINITION_CONTEXT('part definition',#6442,'design');
#6383=PRODUCT_DEFINITION('Cage','Cage',#6408,#6365);
#6408=PRODUCT_DEFINITION_FORMATION('',$,#6461);
#6442=APPLICATION_CONTEXT(
'Core Data for Automotive Mechanical Design Process');
#6443=PRODUCT_CONTEXT('part definition',#6442,'mechanical');
#6461=PRODUCT('Cage','Cage','Cage',(#6443));
#6532=COLOUR_RGB('Grey',0.48,0.52,0.57);
#6533=FILL_AREA_STYLE_COLOUR('',#6532);
#6534=FILL_AREA_STYLE('',(#6533));
#6535=SURFACE_STYLE_FILL_AREA(#6534);
#6536=SURFACE_SIDE_STYLE('',(#6535));
#6537=SURFACE_STYLE_USAGE(.BOTH.,#6536);
#6538=PRESENTATION_STYLE_ASSIGNMENT((#6537));
ENDSEC;
END-ISO-10303-21;
